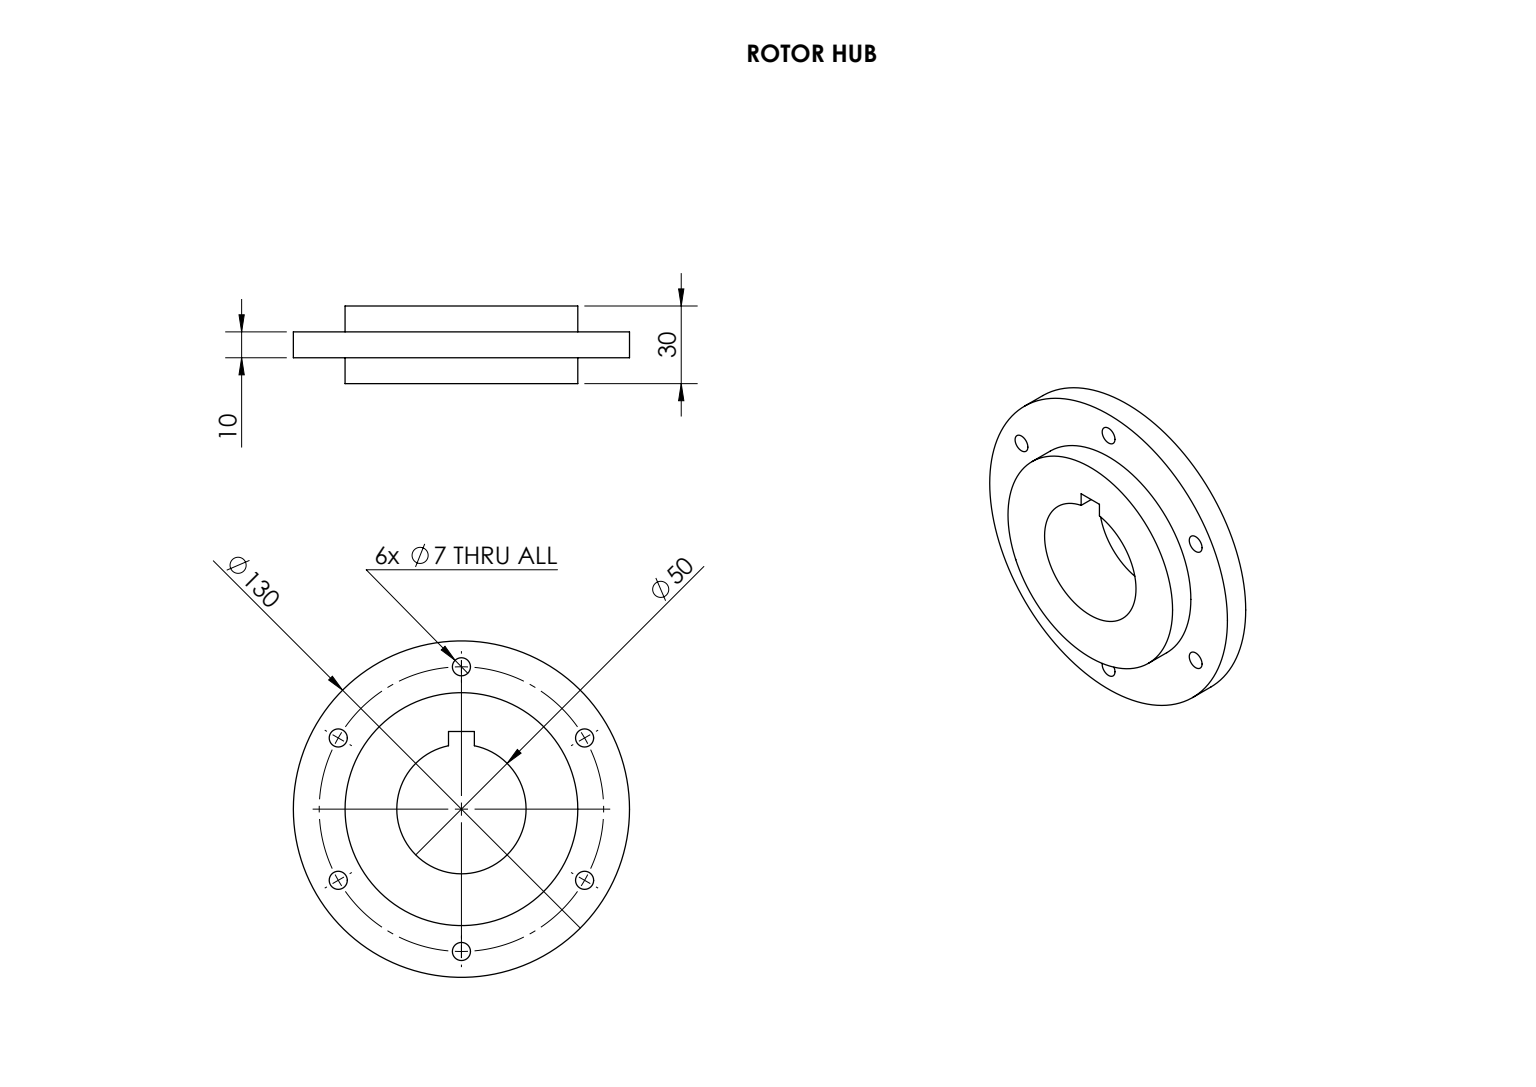
ISO-10303-21;
HEADER;
FILE_DESCRIPTION (('STEP AP214'),
    '1' );
FILE_NAME ('rotor hub.step',
    '2026-09-21T15:58:29',
    ( '' ),
    ( '' ),
    'SwSTEP 2.0',
    'SolidWorks 2026',
    '' );
FILE_SCHEMA (( 'AUTOMOTIVE_DESIGN' ));
ENDSEC;

DATA;
#23=ORIENTED_EDGE ( 'NONE', *, *, #7418, .F. ) ;
#62=ORIENTED_EDGE ( 'NONE', *, *, #28158, .F. ) ;
#132=EDGE_LOOP ( 'NONE', ( #17716, #15446, #15780, #32806 ) ) ;
#135=DIRECTION ( 'NONE',  ( 1.000000000000000000, 0.000000000000000000, 0.000000000000000000 ) ) ;
#170=EDGE_CURVE ( 'NONE', #35280, #21315, #27084, .T. ) ;
#178=CARTESIAN_POINT ( 'NONE',  ( 0.000000000000000000, 0.000000000000000000, -15.00000000000000000 ) ) ;
#209=EDGE_LOOP ( 'NONE', ( #36772, #14646 ) ) ;
#216=ORIENTED_EDGE ( 'NONE', *, *, #28158, .T. ) ;
#229=CARTESIAN_POINT ( 'NONE',  ( 0.000000000000000000, -55.00000000000000000, 5.000000000000000888 ) ) ;
#247=CARTESIAN_POINT ( 'NONE',  ( -47.63139720814438505, -27.49999999999955591, -5.000000000000000888 ) ) ;
#391=ORIENTED_EDGE ( 'NONE', *, *, #32304, .T. ) ;
#413=STYLED_ITEM ( 'NONE', ( #19324 ), #17045 ) ;
#421=ORIENTED_EDGE ( 'NONE', *, *, #12604, .F. ) ;
#524=VECTOR ( 'NONE', #22950, 1000.000000000000000 ) ;
#536=EDGE_CURVE ( 'NONE', #19811, #13357, #11783, .T. ) ;
#674=DIRECTION ( 'NONE',  ( 0.000000000000000000, 0.000000000000000000, 1.000000000000000000 ) ) ;
#679=EDGE_CURVE ( 'NONE', #31822, #13995, #25431, .T. ) ;
#680=FACE_OUTER_BOUND ( 'NONE', #28882, .T. ) ;
#743=DIRECTION ( 'NONE',  ( -1.000000000000000000, 0.000000000000000000, 0.000000000000000000 ) ) ;
#764=CARTESIAN_POINT ( 'NONE',  ( -5.000000000000000000, 24.49489742783178414, 15.00000000000000000 ) ) ;
#824=LINE ( 'NONE', #20902, #10192 ) ;
#838=DIRECTION ( 'NONE',  ( -1.000000000000000000, 0.000000000000000000, 0.000000000000000000 ) ) ;
#971=CARTESIAN_POINT ( 'NONE',  ( -45.00000000000000000, 0.000000000000000000, -15.00000000000000000 ) ) ;
#1002=EDGE_LOOP ( 'NONE', ( #30017, #31364, #12211, #17517 ) ) ;
#1009=ORIENTED_EDGE ( 'NONE', *, *, #1750, .F. ) ;
#1040=CARTESIAN_POINT ( 'NONE',  ( 0.000000000000000000, 55.00000000000000000, -15.00000000000000000 ) ) ;
#1174=DIRECTION ( 'NONE',  ( 1.000000000000000000, 0.000000000000000000, 0.000000000000000000 ) ) ;
#1179=DIRECTION ( 'NONE',  ( 1.000000000000000000, 0.000000000000000000, 0.000000000000000000 ) ) ;
#1187=ORIENTED_EDGE ( 'NONE', *, *, #32304, .F. ) ;
#1244=FACE_BOUND ( 'NONE', #25604, .T. ) ;
#1245=SURFACE_STYLE_USAGE ( .BOTH. , #13045 ) ;
#1283=ORIENTED_EDGE ( 'NONE', *, *, #14933, .F. ) ;
#1311=ORIENTED_EDGE ( 'NONE', *, *, #7418, .T. ) ;
#1329=ADVANCED_FACE ( 'NONE', ( #32145 ), #4233, .F. ) ;
#1402=FACE_OUTER_BOUND ( 'NONE', #32272, .T. ) ;
#1408=ORIENTED_EDGE ( 'NONE', *, *, #15156, .T. ) ;
#1419=PRESENTATION_STYLE_ASSIGNMENT (( #1245 ) ) ;
#1420=EDGE_LOOP ( 'NONE', ( #24774, #7913, #20426, #34060 ) ) ;
#1425=CARTESIAN_POINT ( 'NONE',  ( -4.999999999999999112, 24.49489742783178059, 15.00000000000000000 ) ) ;
#1484=VECTOR ( 'NONE', #4946, 1000.000000000000000 ) ;
#1578=CARTESIAN_POINT ( 'NONE',  ( -5.000000000000000000, 30.00000000000000355, -15.00000000000000000 ) ) ;
#1591=ORIENTED_EDGE ( 'NONE', *, *, #11289, .F. ) ;
#1630=( GEOMETRIC_REPRESENTATION_CONTEXT ( 3 ) GLOBAL_UNCERTAINTY_ASSIGNED_CONTEXT ( ( #8434 ) ) GLOBAL_UNIT_ASSIGNED_CONTEXT ( ( #30742, #18767, #10319 ) ) REPRESENTATION_CONTEXT ( 'NONE', 'WORKASPACE' ) );
#1650=PLANE ( 'NONE',  #21521 ) ;
#1656=DIRECTION ( 'NONE',  ( 0.000000000000000000, 0.000000000000000000, 1.000000000000000000 ) ) ;
#1674=VECTOR ( 'NONE', #17302, 1000.000000000000000 ) ;
#1750=EDGE_CURVE ( 'NONE', #19879, #6148, #24587, .T. ) ;
#1814=CARTESIAN_POINT ( 'NONE',  ( 0.000000000000000000, -55.00000000000000000, -5.000000000000000888 ) ) ;
#1817=CARTESIAN_POINT ( 'NONE',  ( -47.63139720814438505, -27.49999999999955591, -15.00000000000000000 ) ) ;
#1820=VERTEX_POINT ( 'NONE', #31898 ) ;
#1862=DIRECTION ( 'NONE',  ( -1.000000000000000000, 0.000000000000000000, 0.000000000000000000 ) ) ;
#1888=FILL_AREA_STYLE ('',( #4896 ) ) ;
#1909=DIRECTION ( 'NONE',  ( -0.000000000000000000, -0.000000000000000000, 1.000000000000000000 ) ) ;
#2009=DIRECTION ( 'NONE',  ( 1.000000000000000000, 0.000000000000000000, -0.000000000000000000 ) ) ;
#2013=PLANE ( 'NONE',  #17910 ) ;
#2051=CIRCLE ( 'NONE', #23596, 45.00000000000000000 ) ;
#2096=EDGE_LOOP ( 'NONE', ( #27715, #24224, #28476, #9643 ) ) ;
#2103=ORIENTED_EDGE ( 'NONE', *, *, #20963, .T. ) ;
#2104=AXIS2_PLACEMENT_3D ( 'NONE', #2399, #16446, #36696 ) ;
#2150=DIRECTION ( 'NONE',  ( 1.000000000000000000, 0.000000000000000000, 0.000000000000000000 ) ) ;
#2202=DIRECTION ( 'NONE',  ( 0.000000000000000000, 0.000000000000000000, 1.000000000000000000 ) ) ;
#2296=ORIENTED_EDGE ( 'NONE', *, *, #19769, .T. ) ;
#2368=EDGE_CURVE ( 'NONE', #24370, #17590, #4662, .T. ) ;
#2372=VERTEX_POINT ( 'NONE', #14928 ) ;
#2375=EDGE_CURVE ( 'NONE', #2372, #1820, #22821, .T. ) ;
#2399=CARTESIAN_POINT ( 'NONE',  ( 0.000000000000000000, 0.000000000000000000, 15.00000000000000000 ) ) ;
#2480=FACE_BOUND ( 'NONE', #36377, .T. ) ;
#2506=DIRECTION ( 'NONE',  ( -1.000000000000000000, 0.000000000000000000, 0.000000000000000000 ) ) ;
#2557=EDGE_CURVE ( 'NONE', #25534, #2372, #24485, .T. ) ;
#2569=ADVANCED_FACE ( 'NONE', ( #1402 ), #12824, .F. ) ;
#2602=VECTOR ( 'NONE', #10246, 1000.000000000000000 ) ;
#2627=( GEOMETRIC_REPRESENTATION_CONTEXT ( 3 ) GLOBAL_UNCERTAINTY_ASSIGNED_CONTEXT ( ( #4325 ) ) GLOBAL_UNIT_ASSIGNED_CONTEXT ( ( #7421, #26546, #3684 ) ) REPRESENTATION_CONTEXT ( 'NONE', 'WORKASPACE' ) );
#2635=ORIENTED_EDGE ( 'NONE', *, *, #31325, .F. ) ;
#2639=DIRECTION ( 'NONE',  ( -0.000000000000000000, -0.000000000000000000, -1.000000000000000000 ) ) ;
#2674=PRODUCT_DEFINITION ( 'UNKNOWN', '', #29130, #14421 ) ;
#2703=CYLINDRICAL_SURFACE ( 'NONE', #25764, 3.500000000000003109 ) ;
#2741=DIRECTION ( 'NONE',  ( 1.000000000000000000, 0.000000000000000000, 0.000000000000000000 ) ) ;
#2758=EDGE_CURVE ( 'NONE', #24629, #10920, #12743, .T. ) ;
#2891=VECTOR ( 'NONE', #27089, 1000.000000000000000 ) ;
#2947=DIRECTION ( 'NONE',  ( 1.000000000000000000, 0.000000000000000000, 0.000000000000000000 ) ) ;
#2982=CIRCLE ( 'NONE', #8366, 3.500000000000003109 ) ;
#3001=ORIENTED_EDGE ( 'NONE', *, *, #20598, .F. ) ;
#3037=ORIENTED_EDGE ( 'NONE', *, *, #5291, .T. ) ;
#3041=FACE_BOUND ( 'NONE', #30009, .T. ) ;
#3057=CARTESIAN_POINT ( 'NONE',  ( -51.13139720814438505, -27.49999999999955591, -15.00000000000000000 ) ) ;
#3059=ORIENTED_EDGE ( 'NONE', *, *, #2557, .F. ) ;
#3067=CARTESIAN_POINT ( 'NONE',  ( 44.13139720814418610, 27.49999999999988987, -5.000000000000000888 ) ) ;
#3157=CARTESIAN_POINT ( 'NONE',  ( -25.00000000000000000, 0.000000000000000000, 15.00000000000000000 ) ) ;
#3160=EDGE_CURVE ( 'NONE', #36052, #13357, #33221, .T. ) ;
#3172=EDGE_CURVE ( 'NONE', #35280, #29596, #27218, .T. ) ;
#3174=APPLICATION_CONTEXT ( 'automotive_design' ) ;
#3181=DIRECTION ( 'NONE',  ( 0.000000000000000000, 0.000000000000000000, 1.000000000000000000 ) ) ;
#3198=CARTESIAN_POINT ( 'NONE',  ( -47.63139720814380951, 27.50000000000055422, -5.000000000000000888 ) ) ;
#3241=DIRECTION ( 'NONE',  ( 0.000000000000000000, -0.000000000000000000, -1.000000000000000000 ) ) ;
#3281=EDGE_CURVE ( 'NONE', #17590, #24370, #24061, .T. ) ;
#3324=VERTEX_POINT ( 'NONE', #22732 ) ;
#3335=AXIS2_PLACEMENT_3D ( 'NONE', #13182, #24631, #33228 ) ;
#3356=ADVANCED_FACE ( 'NONE', ( #11815, #16738, #3041, #2480, #5479, #16905, #36978, #34524 ), #8469, .F. ) ;
#3417=DIRECTION ( 'NONE',  ( 1.000000000000000000, 0.000000000000000000, 0.000000000000000000 ) ) ;
#3427=COLOUR_RGB ( '', 0.08235294, 0.09019608, 0.10196078) ;
#3448=VERTEX_POINT ( 'NONE', #6941 ) ;
#3599=DIRECTION ( 'NONE',  ( 0.000000000000000000, 0.000000000000000000, 1.000000000000000000 ) ) ;
#3601=LINE ( 'NONE', #3057, #11251 ) ;
#3608=ORIENTED_EDGE ( 'NONE', *, *, #10532, .F. ) ;
#3673=CARTESIAN_POINT ( 'NONE',  ( -5.000000000000000000, 25.00000000000000000, 15.00000000000000000 ) ) ;
#3684=( NAMED_UNIT ( * ) SI_UNIT ( $, .STERADIAN. ) SOLID_ANGLE_UNIT ( ) );
#3692=CARTESIAN_POINT ( 'NONE',  ( -45.00000000000000000, 0.000000000000000000, 15.00000000000000000 ) ) ;
#3696=EDGE_CURVE ( 'NONE', #24370, #5854, #12082, .T. ) ;
#3717=DIRECTION ( 'NONE',  ( 1.000000000000000000, 0.000000000000000000, 0.000000000000000000 ) ) ;
#3725=DIRECTION ( 'NONE',  ( 0.000000000000000000, 0.000000000000000000, 1.000000000000000000 ) ) ;
#3769=ORIENTED_EDGE ( 'NONE', *, *, #32301, .T. ) ;
#3854=CARTESIAN_POINT ( 'NONE',  ( 0.000000000000000000, 0.000000000000000000, -15.00000000000000000 ) ) ;
#3882=EDGE_CURVE ( 'NONE', #4744, #14689, #24525, .T. ) ;
#3948=AXIS2_PLACEMENT_3D ( 'NONE', #178, #26255, #26610 ) ;
#3959=CIRCLE ( 'NONE', #20729, 3.500000000000003109 ) ;
#4002=VECTOR ( 'NONE', #29085, 1000.000000000000000 ) ;
#4077=EDGE_CURVE ( 'NONE', #3448, #10920, #10594, .T. ) ;
#4084=VECTOR ( 'NONE', #35649, 1000.000000000000000 ) ;
#4133=AXIS2_PLACEMENT_3D ( 'NONE', #9406, #15208, #3417 ) ;
#4185=EDGE_CURVE ( 'NONE', #25427, #11646, #25588, .T. ) ;
#4220=AXIS2_PLACEMENT_3D ( 'NONE', #28699, #9174, #743 ) ;
#4226=LINE ( 'NONE', #10576, #1484 ) ;
#4233=CYLINDRICAL_SURFACE ( 'NONE', #13387, 25.00000000000000000 ) ;
#4250=DIRECTION ( 'NONE',  ( 1.000000000000000000, 0.000000000000000000, 0.000000000000000000 ) ) ;
#4325=UNCERTAINTY_MEASURE_WITH_UNIT (LENGTH_MEASURE( 1.000000000000000082E-05 ), #7421, 'distance_accuracy_value', 'NONE');
#4383=CYLINDRICAL_SURFACE ( 'NONE', #11462, 25.00000000000000000 ) ;
#4432=CARTESIAN_POINT ( 'NONE',  ( 47.63139720814418610, 27.49999999999988987, -15.00000000000000000 ) ) ;
#4440=CARTESIAN_POINT ( 'NONE',  ( 3.500000000000000888, -55.00000000000000000, -15.00000000000000000 ) ) ;
#4478=VERTEX_POINT ( 'NONE', #22181 ) ;
#4500=CIRCLE ( 'NONE', #20064, 3.500000000000000888 ) ;
#4514=EDGE_LOOP ( 'NONE', ( #5305, #3608, #4752, #1408 ) ) ;
#4561=EDGE_CURVE ( 'NONE', #25776, #5222, #16511, .T. ) ;
#4602=ORIENTED_EDGE ( 'NONE', *, *, #13796, .T. ) ;
#4609=DIRECTION ( 'NONE',  ( 0.000000000000000000, 0.000000000000000000, 1.000000000000000000 ) ) ;
#4617=VECTOR ( 'NONE', #35577, 1000.000000000000000 ) ;
#4662=CIRCLE ( 'NONE', #22641, 3.500000000000003109 ) ;
#4744=VERTEX_POINT ( 'NONE', #9944 ) ;
#4752=ORIENTED_EDGE ( 'NONE', *, *, #35183, .T. ) ;
#4757=ORIENTED_EDGE ( 'NONE', *, *, #10532, .T. ) ;
#4765=FACE_OUTER_BOUND ( 'NONE', #4997, .T. ) ;
#4783=EDGE_CURVE ( 'NONE', #30464, #18023, #13532, .T. ) ;
#4848=FACE_BOUND ( 'NONE', #18275, .T. ) ;
#4860=AXIS2_PLACEMENT_3D ( 'NONE', #14407, #26015, #135 ) ;
#4896=FILL_AREA_STYLE_COLOUR ( '', #3427 ) ;
#4915=DIRECTION ( 'NONE',  ( 1.000000000000000000, 0.000000000000000000, 0.000000000000000000 ) ) ;
#4921=DIRECTION ( 'NONE',  ( 1.000000000000000000, 0.000000000000000000, 0.000000000000000000 ) ) ;
#4946=DIRECTION ( 'NONE',  ( -0.000000000000000000, -0.000000000000000000, 1.000000000000000000 ) ) ;
#4997=EDGE_LOOP ( 'NONE', ( #31009, #30211, #12672, #1591 ) ) ;
#4998=ORIENTED_EDGE ( 'NONE', *, *, #3172, .T. ) ;
#5065=SHAPE_REPRESENTATION_RELATIONSHIP ( 'NONE' , 'NONE' ,  #33474, #17045 ) ;
#5086=CARTESIAN_POINT ( 'NONE',  ( 25.00000000000000000, 3.061616997868383043E-15, 15.00000000000000000 ) ) ;
#5210=CARTESIAN_POINT ( 'NONE',  ( 0.000000000000000000, 0.000000000000000000, 5.000000000000000000 ) ) ;
#5222=VERTEX_POINT ( 'NONE', #26891 ) ;
#5259=EDGE_CURVE ( 'NONE', #10522, #31822, #7379, .T. ) ;
#5275=ORIENTED_EDGE ( 'NONE', *, *, #12604, .T. ) ;
#5291=EDGE_CURVE ( 'NONE', #31944, #11785, #16372, .T. ) ;
#5305=ORIENTED_EDGE ( 'NONE', *, *, #26190, .F. ) ;
#5392=CARTESIAN_POINT ( 'NONE',  ( -5.000000000000000000, 30.00000000000000355, -15.00000000000000000 ) ) ;
#5416=AXIS2_PLACEMENT_3D ( 'NONE', #229, #23120, #28913 ) ;
#5479=FACE_BOUND ( 'NONE', #29963, .T. ) ;
#5592=DIRECTION ( 'NONE',  ( -0.000000000000000000, -0.000000000000000000, 1.000000000000000000 ) ) ;
#5694=AXIS2_PLACEMENT_3D ( 'NONE', #32993, #7307, #13120 ) ;
#5730=CARTESIAN_POINT ( 'NONE',  ( 0.000000000000000000, 0.000000000000000000, 15.00000000000000000 ) ) ;
#5761=CARTESIAN_POINT ( 'NONE',  ( -51.13139720814380951, 27.50000000000055422, -5.000000000000000888 ) ) ;
#5846=DIRECTION ( 'NONE',  ( 0.000000000000000000, 0.000000000000000000, 1.000000000000000000 ) ) ;
#5854=VERTEX_POINT ( 'NONE', #28984 ) ;
#5899=CARTESIAN_POINT ( 'NONE',  ( 5.000000000000000000, 24.49489742783178414, -15.00000000000000000 ) ) ;
#5910=( LENGTH_UNIT ( ) NAMED_UNIT ( * ) SI_UNIT ( .MILLI., .METRE. ) );
#6012=ORIENTED_EDGE ( 'NONE', *, *, #2758, .F. ) ;
#6044=DIRECTION ( 'NONE',  ( 1.000000000000000000, 0.000000000000000000, 0.000000000000000000 ) ) ;
#6073=VECTOR ( 'NONE', #25857, 1000.000000000000000 ) ;
#6092=CARTESIAN_POINT ( 'NONE',  ( -65.00000000000000000, 0.000000000000000000, 5.000000000000000000 ) ) ;
#6148=VERTEX_POINT ( 'NONE', #32743 ) ;
#6412=DIRECTION ( 'NONE',  ( 1.000000000000000000, 0.000000000000000000, 0.000000000000000000 ) ) ;
#6432=AXIS2_PLACEMENT_3D ( 'NONE', #6988, #10187, #29863 ) ;
#6489=ORIENTED_EDGE ( 'NONE', *, *, #19945, .T. ) ;
#6491=DIRECTION ( 'NONE',  ( 1.000000000000000000, 0.000000000000000000, 0.000000000000000000 ) ) ;
#6588=EDGE_CURVE ( 'NONE', #3448, #14395, #16778, .T. ) ;
#6795=COLOUR_RGB ( '', 0.08235294, 0.09019608, 0.10196078) ;
#6813=FACE_OUTER_BOUND ( 'NONE', #132, .T. ) ;
#6842=DIRECTION ( 'NONE',  ( 1.000000000000000000, 0.000000000000000000, 0.000000000000000000 ) ) ;
#6873=EDGE_CURVE ( 'NONE', #11785, #11646, #22180, .T. ) ;
#6941=CARTESIAN_POINT ( 'NONE',  ( 51.13139720814400846, -27.50000000000022737, -5.000000000000000888 ) ) ;
#6956=DIRECTION ( 'NONE',  ( 1.000000000000000000, 0.000000000000000000, 0.000000000000000000 ) ) ;
#6978=DIRECTION ( 'NONE',  ( 0.000000000000000000, 0.000000000000000000, 1.000000000000000000 ) ) ;
#6986=DIRECTION ( 'NONE',  ( 1.000000000000000000, 0.000000000000000000, 0.000000000000000000 ) ) ;
#6988=CARTESIAN_POINT ( 'NONE',  ( 0.000000000000000000, 0.000000000000000000, -5.000000000000000000 ) ) ;
#7014=DIRECTION ( 'NONE',  ( -1.000000000000000000, 0.000000000000000000, 0.000000000000000000 ) ) ;
#7071=CYLINDRICAL_SURFACE ( 'NONE', #28018, 3.500000000000003109 ) ;
#7095=CARTESIAN_POINT ( 'NONE',  ( -47.63139720814380951, 27.50000000000055422, -15.00000000000000000 ) ) ;
#7159=AXIS2_PLACEMENT_3D ( 'NONE', #5210, #1656, #27882 ) ;
#7183=CIRCLE ( 'NONE', #28131, 45.00000000000000000 ) ;
#7246=ORIENTED_EDGE ( 'NONE', *, *, #34520, .T. ) ;
#7307=DIRECTION ( 'NONE',  ( 0.000000000000000000, 0.000000000000000000, 1.000000000000000000 ) ) ;
#7321=UNCERTAINTY_MEASURE_WITH_UNIT (LENGTH_MEASURE( 1.000000000000000082E-05 ), #5910, 'distance_accuracy_value', 'NONE');
#7379=LINE ( 'NONE', #12228, #18359 ) ;
#7407=DIRECTION ( 'NONE',  ( 0.000000000000000000, 0.000000000000000000, -1.000000000000000000 ) ) ;
#7418=EDGE_CURVE ( 'NONE', #31822, #2372, #16028, .T. ) ;
#7421=( LENGTH_UNIT ( ) NAMED_UNIT ( * ) SI_UNIT ( .MILLI., .METRE. ) );
#7528=DIRECTION ( 'NONE',  ( -0.000000000000000000, 0.000000000000000000, 1.000000000000000000 ) ) ;
#7575=AXIS2_PLACEMENT_3D ( 'NONE', #24426, #6978, #1179 ) ;
#7647=CYLINDRICAL_SURFACE ( 'NONE', #2104, 45.00000000000000000 ) ;
#7709=CYLINDRICAL_SURFACE ( 'NONE', #21484, 25.00000000000000000 ) ;
#7740=CARTESIAN_POINT ( 'NONE',  ( 0.000000000000000000, 55.00000000000000000, -5.000000000000000888 ) ) ;
#7764=CARTESIAN_POINT ( 'NONE',  ( 5.000000000000000000, 24.49489742783178414, 15.00000000000000000 ) ) ;
#7773=AXIS2_PLACEMENT_3D ( 'NONE', #7095, #12882, #18542 ) ;
#7830=DIRECTION ( 'NONE',  ( 0.000000000000000000, 0.000000000000000000, 1.000000000000000000 ) ) ;
#7859=EDGE_CURVE ( 'NONE', #11646, #11785, #16773, .T. ) ;
#7913=ORIENTED_EDGE ( 'NONE', *, *, #20003, .T. ) ;
#7971=DIRECTION ( 'NONE',  ( 1.000000000000000000, 0.000000000000000000, 0.000000000000000000 ) ) ;
#7994=DIRECTION ( 'NONE',  ( 1.000000000000000000, 0.000000000000000000, 0.000000000000000000 ) ) ;
#8033=AXIS2_PLACEMENT_3D ( 'NONE', #20629, #3599, #6044 ) ;
#8044=EDGE_CURVE ( 'NONE', #21315, #26861, #31149, .T. ) ;
#8098=DIRECTION ( 'NONE',  ( -0.000000000000000000, 0.000000000000000000, 1.000000000000000000 ) ) ;
#8104=AXIS2_PLACEMENT_3D ( 'NONE', #35168, #20703, #9655 ) ;
#8113=ADVANCED_FACE ( 'NONE', ( #20604 ), #17443, .T. ) ;
#8219=CLOSED_SHELL ( 'NONE', ( #14021, #22878, #20690, #14478, #10904, #2569, #18517, #22051, #1329, #28849, #22091, #35522, #14922, #15263, #17435, #11394, #34187, #8591, #30019, #13997, #3356, #8113, #17566, #19990, #13254, #27020, #30785, #29252 ) ) ;
#8250=CARTESIAN_POINT ( 'NONE',  ( 3.500000000000000888, 55.00000000000000000, 5.000000000000000888 ) ) ;
#8366=AXIS2_PLACEMENT_3D ( 'NONE', #18502, #10408, #4250 ) ;
#8384=DIRECTION ( 'NONE',  ( 0.000000000000000000, 0.000000000000000000, 1.000000000000000000 ) ) ;
#8434=UNCERTAINTY_MEASURE_WITH_UNIT (LENGTH_MEASURE( 1.000000000000000082E-05 ), #30742, 'distance_accuracy_value', 'NONE');
#8469=PLANE ( 'NONE',  #19276 ) ;
#8537=EDGE_CURVE ( 'NONE', #25534, #35280, #16235, .T. ) ;
#8591=ADVANCED_FACE ( 'NONE', ( #34836 ), #9132, .T. ) ;
#8630=LINE ( 'NONE', #28317, #33793 ) ;
#8642=ORIENTED_EDGE ( 'NONE', *, *, #8739, .T. ) ;
#8658=EDGE_LOOP ( 'NONE', ( #27899, #10390 ) ) ;
#8702=AXIS2_PLACEMENT_3D ( 'NONE', #27436, #30054, #24243 ) ;
#8722=CARTESIAN_POINT ( 'NONE',  ( 25.00000000000000000, 3.061616997868383043E-15, -15.00000000000000000 ) ) ;
#8739=EDGE_CURVE ( 'NONE', #13777, #14961, #20102, .T. ) ;
#8762=ORIENTED_EDGE ( 'NONE', *, *, #19494, .T. ) ;
#8880=AXIS2_PLACEMENT_3D ( 'NONE', #15616, #13335, #4915 ) ;
#8896=CARTESIAN_POINT ( 'NONE',  ( 0.000000000000000000, 0.000000000000000000, 0.000000000000000000 ) ) ;
#8913=DIRECTION ( 'NONE',  ( -0.000000000000000000, -0.000000000000000000, -1.000000000000000000 ) ) ;
#8924=ORIENTED_EDGE ( 'NONE', *, *, #20598, .T. ) ;
#9008=ORIENTED_EDGE ( 'NONE', *, *, #27912, .F. ) ;
#9095=ORIENTED_EDGE ( 'NONE', *, *, #32301, .F. ) ;
#9111=CARTESIAN_POINT ( 'NONE',  ( 0.000000000000000000, 0.000000000000000000, -15.00000000000000000 ) ) ;
#9128=AXIS2_PLACEMENT_3D ( 'NONE', #16301, #13465, #1862 ) ;
#9132=PLANE ( 'NONE',  #23422 ) ;
#9174=DIRECTION ( 'NONE',  ( -0.000000000000000000, -0.000000000000000000, -1.000000000000000000 ) ) ;
#9226=ORIENTED_EDGE ( 'NONE', *, *, #8044, .T. ) ;
#9264=DIRECTION ( 'NONE',  ( -0.000000000000000000, -0.000000000000000000, 1.000000000000000000 ) ) ;
#9406=CARTESIAN_POINT ( 'NONE',  ( 0.000000000000000000, 0.000000000000000000, 5.000000000000000000 ) ) ;
#9504=DIRECTION ( 'NONE',  ( 1.000000000000000000, 0.000000000000000000, 0.000000000000000000 ) ) ;
#9585=EDGE_CURVE ( 'NONE', #20938, #36052, #27332, .T. ) ;
#9595=LINE ( 'NONE', #23647, #34378 ) ;
#9643=ORIENTED_EDGE ( 'NONE', *, *, #7859, .T. ) ;
#9655=DIRECTION ( 'NONE',  ( 1.000000000000000000, 0.000000000000000000, 0.000000000000000000 ) ) ;
#9676=ORIENTED_EDGE ( 'NONE', *, *, #30500, .T. ) ;
#9688=ORIENTED_EDGE ( 'NONE', *, *, #13106, .F. ) ;
#9800=ORIENTED_EDGE ( 'NONE', *, *, #2758, .T. ) ;
#9836=CARTESIAN_POINT ( 'NONE',  ( 5.000000000000000000, 25.00000000000000000, -15.00000000000000000 ) ) ;
#9907=CARTESIAN_POINT ( 'NONE',  ( 45.00000000000000711, 5.510910596163091133E-15, 5.000000000000000000 ) ) ;
#9930=DIRECTION ( 'NONE',  ( 0.000000000000000000, -0.000000000000000000, 1.000000000000000000 ) ) ;
#9944=CARTESIAN_POINT ( 'NONE',  ( 65.00000000000000000, 7.960204194457797252E-15, -5.000000000000000000 ) ) ;
#9946=ORIENTED_EDGE ( 'NONE', *, *, #13106, .T. ) ;
#10099=ORIENTED_EDGE ( 'NONE', *, *, #4077, .T. ) ;
#10187=DIRECTION ( 'NONE',  ( 0.000000000000000000, 0.000000000000000000, 1.000000000000000000 ) ) ;
#10192=VECTOR ( 'NONE', #12237, 1000.000000000000000 ) ;
#10222=PLANE ( 'NONE',  #30953 ) ;
#10246=DIRECTION ( 'NONE',  ( -0.000000000000000000, 1.000000000000000000, 0.000000000000000000 ) ) ;
#10319=( NAMED_UNIT ( * ) SI_UNIT ( $, .STERADIAN. ) SOLID_ANGLE_UNIT ( ) );
#10363=EDGE_LOOP ( 'NONE', ( #34270, #9226, #62, #34153 ) ) ;
#10390=ORIENTED_EDGE ( 'NONE', *, *, #2368, .T. ) ;
#10399=PRODUCT ( 'rotor hub', 'rotor hub', '', ( #12666 ) ) ;
#10408=DIRECTION ( 'NONE',  ( 0.000000000000000000, 0.000000000000000000, 1.000000000000000000 ) ) ;
#10450=DIRECTION ( 'NONE',  ( 1.000000000000000000, 0.000000000000000000, -0.000000000000000000 ) ) ;
#10522=VERTEX_POINT ( 'NONE', #18345 ) ;
#10532=EDGE_CURVE ( 'NONE', #14697, #30372, #16441, .T. ) ;
#10538=FACE_OUTER_BOUND ( 'NONE', #16439, .T. ) ;
#10576=CARTESIAN_POINT ( 'NONE',  ( -3.500000000000000888, -55.00000000000000000, -15.00000000000000000 ) ) ;
#10594=LINE ( 'NONE', #16951, #19699 ) ;
#10610=SHAPE_DEFINITION_REPRESENTATION ( #17857, #33474 ) ;
#10619=EDGE_CURVE ( 'NONE', #25427, #31944, #32622, .T. ) ;
#10656=FACE_OUTER_BOUND ( 'NONE', #13476, .T. ) ;
#10705=SURFACE_SIDE_STYLE ('',( #13492 ) ) ;
#10806=DIRECTION ( 'NONE',  ( 1.000000000000000000, 0.000000000000000000, 0.000000000000000000 ) ) ;
#10836=FACE_OUTER_BOUND ( 'NONE', #29415, .T. ) ;
#10904=ADVANCED_FACE ( 'NONE', ( #4765 ), #12619, .F. ) ;
#10920=VERTEX_POINT ( 'NONE', #35514 ) ;
#10951=CARTESIAN_POINT ( 'NONE',  ( 47.63139720814418610, 27.49999999999988987, -5.000000000000000888 ) ) ;
#11129=EDGE_CURVE ( 'NONE', #10522, #25534, #14645, .T. ) ;
#11189=EDGE_CURVE ( 'NONE', #20938, #19811, #3601, .T. ) ;
#11236=DIRECTION ( 'NONE',  ( 0.000000000000000000, 0.000000000000000000, 1.000000000000000000 ) ) ;
#11251=VECTOR ( 'NONE', #31523, 1000.000000000000000 ) ;
#11254=ORIENTED_EDGE ( 'NONE', *, *, #36027, .T. ) ;
#11257=EDGE_LOOP ( 'NONE', ( #13857, #17632, #5275, #9946 ) ) ;
#11289=EDGE_CURVE ( 'NONE', #4478, #25776, #27394, .T. ) ;
#11337=FACE_OUTER_BOUND ( 'NONE', #11456, .T. ) ;
#11394=ADVANCED_FACE ( 'NONE', ( #33760 ), #7709, .F. ) ;
#11437=CARTESIAN_POINT ( 'NONE',  ( 0.000000000000000000, 0.000000000000000000, 5.000000000000000000 ) ) ;
#11441=DIRECTION ( 'NONE',  ( 1.000000000000000000, 0.000000000000000000, 0.000000000000000000 ) ) ;
#11442=ORIENTED_EDGE ( 'NONE', *, *, #12384, .F. ) ;
#11454=DIRECTION ( 'NONE',  ( 0.000000000000000000, 0.000000000000000000, 1.000000000000000000 ) ) ;
#11456=EDGE_LOOP ( 'NONE', ( #23334, #18031, #9800, #33838 ) ) ;
#11462=AXIS2_PLACEMENT_3D ( 'NONE', #35898, #32686, #7014 ) ;
#11618=CARTESIAN_POINT ( 'NONE',  ( -5.000000000000000000, 30.00000000000000355, -15.00000000000000000 ) ) ;
#11646=VERTEX_POINT ( 'NONE', #29410 ) ;
#11741=AXIS2_PLACEMENT_3D ( 'NONE', #247, #34591, #29121 ) ;
#11752=ORIENTED_EDGE ( 'NONE', *, *, #2375, .T. ) ;
#11783=CIRCLE ( 'NONE', #32758, 3.500000000000003109 ) ;
#11785=VERTEX_POINT ( 'NONE', #9907 ) ;
#11815=FACE_BOUND ( 'NONE', #8658, .T. ) ;
#11961=AXIS2_PLACEMENT_3D ( 'NONE', #1814, #13241, #36119 ) ;
#12082=LINE ( 'NONE', #23543, #6073 ) ;
#12211=ORIENTED_EDGE ( 'NONE', *, *, #3160, .T. ) ;
#12228=CARTESIAN_POINT ( 'NONE',  ( -5.000000000000000000, 25.00000000000000000, -15.00000000000000000 ) ) ;
#12237=DIRECTION ( 'NONE',  ( -0.000000000000000000, -0.000000000000000000, -1.000000000000000000 ) ) ;
#12306=AXIS2_PLACEMENT_3D ( 'NONE', #10951, #4609, #22907 ) ;
#12336=CIRCLE ( 'NONE', #7575, 3.500000000000003109 ) ;
#12384=EDGE_CURVE ( 'NONE', #21315, #22186, #25749, .T. ) ;
#12405=EDGE_CURVE ( 'NONE', #18518, #21193, #14976, .T. ) ;
#12446=AXIS2_PLACEMENT_3D ( 'NONE', #1040, #32916, #6491 ) ;
#12486=AXIS2_PLACEMENT_3D ( 'NONE', #7740, #30604, #4921 ) ;
#12574=AXIS2_PLACEMENT_3D ( 'NONE', #11437, #3181, #17802 ) ;
#12604=EDGE_CURVE ( 'NONE', #25787, #14689, #824, .T. ) ;
#12619=CYLINDRICAL_SURFACE ( 'NONE', #8702, 3.500000000000003109 ) ;
#12657=ORIENTED_EDGE ( 'NONE', *, *, #9585, .F. ) ;
#12666=PRODUCT_CONTEXT ( 'NONE', #3174, 'mechanical' ) ;
#12672=ORIENTED_EDGE ( 'NONE', *, *, #16828, .T. ) ;
#12674=DIRECTION ( 'NONE',  ( 0.000000000000000000, -0.000000000000000000, 1.000000000000000000 ) ) ;
#12743=CIRCLE ( 'NONE', #22964, 3.500000000000003109 ) ;
#12808=AXIS2_PLACEMENT_3D ( 'NONE', #21595, #33395, #6956 ) ;
#12818=DIRECTION ( 'NONE',  ( -0.000000000000000000, -0.000000000000000000, -1.000000000000000000 ) ) ;
#12824=CYLINDRICAL_SURFACE ( 'NONE', #12446, 3.500000000000000888 ) ;
#12882=DIRECTION ( 'NONE',  ( -0.000000000000000000, -0.000000000000000000, 1.000000000000000000 ) ) ;
#12887=CARTESIAN_POINT ( 'NONE',  ( -3.500000000000000888, 55.00000000000000000, 5.000000000000000888 ) ) ;
#12924=VERTEX_POINT ( 'NONE', #5899 ) ;
#13017=ORIENTED_EDGE ( 'NONE', *, *, #15156, .F. ) ;
#13030=VECTOR ( 'NONE', #24746, 1000.000000000000000 ) ;
#13043=CIRCLE ( 'NONE', #6432, 65.00000000000000000 ) ;
#13045=SURFACE_SIDE_STYLE ('',( #35749 ) ) ;
#13052=FACE_OUTER_BOUND ( 'NONE', #27825, .T. ) ;
#13072=DIRECTION ( 'NONE',  ( 1.000000000000000000, 0.000000000000000000, 0.000000000000000000 ) ) ;
#13079=AXIS2_PLACEMENT_3D ( 'NONE', #27365, #9930, #33167 ) ;
#13106=EDGE_CURVE ( 'NONE', #14689, #4744, #13043, .T. ) ;
#13119=AXIS2_PLACEMENT_3D ( 'NONE', #23033, #11236, #22684 ) ;
#13120=DIRECTION ( 'NONE',  ( 1.000000000000000000, 0.000000000000000000, 0.000000000000000000 ) ) ;
#13174=CARTESIAN_POINT ( 'NONE',  ( -44.13139720814437794, -27.49999999999955591, -15.00000000000000000 ) ) ;
#13182=CARTESIAN_POINT ( 'NONE',  ( 47.63139720814418610, 27.49999999999988987, 5.000000000000000888 ) ) ;
#13203=CARTESIAN_POINT ( 'NONE',  ( 47.63139720814400846, -27.50000000000022737, -5.000000000000000888 ) ) ;
#13216=ORIENTED_EDGE ( 'NONE', *, *, #19835, .T. ) ;
#13238=DIRECTION ( 'NONE',  ( -0.000000000000000000, -0.000000000000000000, 1.000000000000000000 ) ) ;
#13241=DIRECTION ( 'NONE',  ( 0.000000000000000000, 0.000000000000000000, 1.000000000000000000 ) ) ;
#13254=ADVANCED_FACE ( 'NONE', ( #10538 ), #21983, .F. ) ;
#13268=EDGE_CURVE ( 'NONE', #3324, #24335, #16104, .T. ) ;
#13292=DIRECTION ( 'NONE',  ( 0.000000000000000000, 0.000000000000000000, 1.000000000000000000 ) ) ;
#13335=DIRECTION ( 'NONE',  ( 0.000000000000000000, 0.000000000000000000, 1.000000000000000000 ) ) ;
#13340=DIRECTION ( 'NONE',  ( 0.000000000000000000, 0.000000000000000000, 1.000000000000000000 ) ) ;
#13357=VERTEX_POINT ( 'NONE', #20443 ) ;
#13358=ORIENTED_EDGE ( 'NONE', *, *, #4783, .F. ) ;
#13379=MECHANICAL_DESIGN_GEOMETRIC_PRESENTATION_REPRESENTATION('',(#26574),#2627);
#13387=AXIS2_PLACEMENT_3D ( 'NONE', #15662, #12818, #838 ) ;
#13396=AXIS2_PLACEMENT_3D ( 'NONE', #36689, #8384, #2741 ) ;
#13439=DIRECTION ( 'NONE',  ( 0.000000000000000000, 0.000000000000000000, 1.000000000000000000 ) ) ;
#13465=DIRECTION ( 'NONE',  ( -0.000000000000000000, -0.000000000000000000, -1.000000000000000000 ) ) ;
#13469=CARTESIAN_POINT ( 'NONE',  ( -51.13139720814438505, -27.49999999999955591, 5.000000000000000888 ) ) ;
#13476=EDGE_LOOP ( 'NONE', ( #31447, #9676 ) ) ;
#13478=EDGE_LOOP ( 'NONE', ( #19906, #35429 ) ) ;
#13492=SURFACE_STYLE_FILL_AREA ( #1888 ) ;
#13532=CIRCLE ( 'NONE', #27907, 45.00000000000000000 ) ;
#13551=DIRECTION ( 'NONE',  ( -0.000000000000000000, -0.000000000000000000, -1.000000000000000000 ) ) ;
#13727=AXIS2_PLACEMENT_3D ( 'NONE', #24282, #24489, #6842 ) ;
#13777=VERTEX_POINT ( 'NONE', #8250 ) ;
#13796=EDGE_CURVE ( 'NONE', #6148, #19879, #35878, .T. ) ;
#13844=EDGE_LOOP ( 'NONE', ( #391, #34050 ) ) ;
#13854=CARTESIAN_POINT ( 'NONE',  ( 5.000000000000000000, 24.49489742783178414, 15.00000000000000000 ) ) ;
#13857=ORIENTED_EDGE ( 'NONE', *, *, #19494, .F. ) ;
#13947=DIRECTION ( 'NONE',  ( -0.000000000000000000, 0.000000000000000000, 1.000000000000000000 ) ) ;
#13995=VERTEX_POINT ( 'NONE', #19105 ) ;
#13997=ADVANCED_FACE ( 'NONE', ( #19274, #30529, #27524, #30131, #27875, #4848, #30690, #16278 ), #1650, .T. ) ;
#14021=ADVANCED_FACE ( 'NONE', ( #10836 ), #32774, .F. ) ;
#14114=AXIS2_PLACEMENT_3D ( 'NONE', #36808, #31538, #2506 ) ;
#14189=ORIENTED_EDGE ( 'NONE', *, *, #3696, .T. ) ;
#14251=CARTESIAN_POINT ( 'NONE',  ( 47.63139720814400846, -27.50000000000022737, -5.000000000000000888 ) ) ;
#14254=DIRECTION ( 'NONE',  ( -1.000000000000000000, 0.000000000000000000, 0.000000000000000000 ) ) ;
#14256=ORIENTED_EDGE ( 'NONE', *, *, #536, .T. ) ;
#14284=DIRECTION ( 'NONE',  ( 1.000000000000000000, 0.000000000000000000, -0.000000000000000000 ) ) ;
#14374=CARTESIAN_POINT ( 'NONE',  ( -5.000000000000000000, 30.00000000000000355, 15.00000000000000000 ) ) ;
#14395=VERTEX_POINT ( 'NONE', #32924 ) ;
#14407=CARTESIAN_POINT ( 'NONE',  ( 0.000000000000000000, 0.000000000000000000, 15.00000000000000000 ) ) ;
#14421=PRODUCT_DEFINITION_CONTEXT ( 'detailed design', #20687, 'design' ) ;
#14451=ORIENTED_EDGE ( 'NONE', *, *, #4561, .T. ) ;
#14465=ORIENTED_EDGE ( 'NONE', *, *, #11129, .T. ) ;
#14478=ADVANCED_FACE ( 'NONE', ( #11337 ), #2703, .F. ) ;
#14544=DIRECTION ( 'NONE',  ( 1.000000000000000000, 0.000000000000000000, 0.000000000000000000 ) ) ;
#14583=EDGE_LOOP ( 'NONE', ( #19347, #1311, #3059, #28096 ) ) ;
#14645=LINE ( 'NONE', #764, #1674 ) ;
#14646=ORIENTED_EDGE ( 'NONE', *, *, #536, .F. ) ;
#14689=VERTEX_POINT ( 'NONE', #19151 ) ;
#14694=( NAMED_UNIT ( * ) PLANE_ANGLE_UNIT ( ) SI_UNIT ( $, .RADIAN. ) );
#14697=VERTEX_POINT ( 'NONE', #22488 ) ;
#14709=ORIENTED_EDGE ( 'NONE', *, *, #2375, .F. ) ;
#14922=ADVANCED_FACE ( 'NONE', ( #18717, #10656 ), #2013, .T. ) ;
#14928=CARTESIAN_POINT ( 'NONE',  ( -5.000000000000000000, 30.00000000000000355, 15.00000000000000000 ) ) ;
#14933=EDGE_CURVE ( 'NONE', #37029, #25787, #29272, .T. ) ;
#14944=PLANE ( 'NONE',  #27519 ) ;
#14961=VERTEX_POINT ( 'NONE', #12887 ) ;
#14976=CIRCLE ( 'NONE', #11961, 3.500000000000000888 ) ;
#15038=CARTESIAN_POINT ( 'NONE',  ( 45.00000000000000000, 5.510910596163089556E-15, 15.00000000000000000 ) ) ;
#15141=DIRECTION ( 'NONE',  ( 1.000000000000000000, 0.000000000000000000, 0.000000000000000000 ) ) ;
#15147=EDGE_LOOP ( 'NONE', ( #14709, #23, #28139, #6489 ) ) ;
#15156=EDGE_CURVE ( 'NONE', #18023, #30464, #7183, .T. ) ;
#15208=DIRECTION ( 'NONE',  ( 0.000000000000000000, 0.000000000000000000, 1.000000000000000000 ) ) ;
#15231=ORIENTED_EDGE ( 'NONE', *, *, #12405, .T. ) ;
#15263=ADVANCED_FACE ( 'NONE', ( #680, #1244 ), #14944, .F. ) ;
#15332=FACE_OUTER_BOUND ( 'NONE', #4514, .T. ) ;
#15397=EDGE_CURVE ( 'NONE', #13357, #19811, #2982, .T. ) ;
#15446=ORIENTED_EDGE ( 'NONE', *, *, #26190, .T. ) ;
#15517=EDGE_CURVE ( 'NONE', #4478, #23649, #34595, .T. ) ;
#15545=ORIENTED_EDGE ( 'NONE', *, *, #8537, .F. ) ;
#15616=CARTESIAN_POINT ( 'NONE',  ( 0.000000000000000000, 0.000000000000000000, 15.00000000000000000 ) ) ;
#15647=DIRECTION ( 'NONE',  ( 1.000000000000000000, 0.000000000000000000, 0.000000000000000000 ) ) ;
#15662=CARTESIAN_POINT ( 'NONE',  ( 0.000000000000000000, 0.000000000000000000, 15.00000000000000000 ) ) ;
#15767=CYLINDRICAL_SURFACE ( 'NONE', #12808, 3.500000000000000888 ) ;
#15780=ORIENTED_EDGE ( 'NONE', *, *, #4783, .T. ) ;
#15963=EDGE_LOOP ( 'NONE', ( #26804, #4998, #2635, #14465 ) ) ;
#16028=LINE ( 'NONE', #1578, #37086 ) ;
#16104=CIRCLE ( 'NONE', #12486, 3.500000000000000888 ) ;
#16111=CARTESIAN_POINT ( 'NONE',  ( -3.500000000000000888, -55.00000000000000000, -5.000000000000000888 ) ) ;
#16120=DIRECTION ( 'NONE',  ( 0.000000000000000000, 0.000000000000000000, 1.000000000000000000 ) ) ;
#16127=CARTESIAN_POINT ( 'NONE',  ( 3.500000000000000888, -55.00000000000000000, -5.000000000000000888 ) ) ;
#16235=CIRCLE ( 'NONE', #4860, 25.00000000000000000 ) ;
#16278=FACE_BOUND ( 'NONE', #28835, .T. ) ;
#16301=CARTESIAN_POINT ( 'NONE',  ( 0.000000000000000000, 0.000000000000000000, 5.000000000000000000 ) ) ;
#16363=EDGE_LOOP ( 'NONE', ( #4757, #29647 ) ) ;
#16372=LINE ( 'NONE', #33448, #23148 ) ;
#16439=EDGE_LOOP ( 'NONE', ( #22401, #26965, #10099, #22300 ) ) ;
#16441=CIRCLE ( 'NONE', #26014, 45.00000000000000000 ) ;
#16446=DIRECTION ( 'NONE',  ( -0.000000000000000000, -0.000000000000000000, -1.000000000000000000 ) ) ;
#16505=DIRECTION ( 'NONE',  ( -0.000000000000000000, -0.000000000000000000, -1.000000000000000000 ) ) ;
#16511=CIRCLE ( 'NONE', #3335, 3.500000000000003109 ) ;
#16527=DIRECTION ( 'NONE',  ( -0.000000000000000000, -0.000000000000000000, -1.000000000000000000 ) ) ;
#16546=ORIENTED_EDGE ( 'NONE', *, *, #27912, .T. ) ;
#16629=CARTESIAN_POINT ( 'NONE',  ( 0.000000000000000000, 55.00000000000000000, 5.000000000000000888 ) ) ;
#16682=LINE ( 'NONE', #13854, #13030 ) ;
#16716=EDGE_CURVE ( 'NONE', #25787, #37029, #22095, .T. ) ;
#16738=FACE_BOUND ( 'NONE', #21324, .T. ) ;
#16773=CIRCLE ( 'NONE', #29333, 45.00000000000000711 ) ;
#16778=CIRCLE ( 'NONE', #36535, 3.500000000000003109 ) ;
#16828=EDGE_CURVE ( 'NONE', #5222, #25776, #3959, .T. ) ;
#16878=CARTESIAN_POINT ( 'NONE',  ( -51.13139720814438505, -27.49999999999955591, -5.000000000000000888 ) ) ;
#16905=FACE_BOUND ( 'NONE', #13844, .T. ) ;
#16951=CARTESIAN_POINT ( 'NONE',  ( 51.13139720814400846, -27.50000000000022737, -15.00000000000000000 ) ) ;
#17023=AXIS2_PLACEMENT_3D ( 'NONE', #32995, #13292, #18745 ) ;
#17045=ADVANCED_BREP_SHAPE_REPRESENTATION ( '', ( #20313, #21385 ), #22589 ) ;
#17183=ORIENTED_EDGE ( 'NONE', *, *, #13796, .F. ) ;
#17186=DIRECTION ( 'NONE',  ( 1.000000000000000000, 0.000000000000000000, 0.000000000000000000 ) ) ;
#17219=EDGE_CURVE ( 'NONE', #18518, #6148, #18516, .T. ) ;
#17237=EDGE_LOOP ( 'NONE', ( #3001, #26636, #26143, #35638 ) ) ;
#17302=DIRECTION ( 'NONE',  ( 0.000000000000000000, 0.000000000000000000, 1.000000000000000000 ) ) ;
#17375=CARTESIAN_POINT ( 'NONE',  ( -47.63139720814380951, 27.50000000000055422, -5.000000000000000888 ) ) ;
#17435=ADVANCED_FACE ( 'NONE', ( #25418 ), #19976, .T. ) ;
#17443=CYLINDRICAL_SURFACE ( 'NONE', #4220, 65.00000000000000000 ) ;
#17469=CARTESIAN_POINT ( 'NONE',  ( 0.000000000000000000, 0.000000000000000000, 15.00000000000000000 ) ) ;
#17517=ORIENTED_EDGE ( 'NONE', *, *, #15397, .T. ) ;
#17566=ADVANCED_FACE ( 'NONE', ( #26518 ), #21460, .F. ) ;
#17590=VERTEX_POINT ( 'NONE', #17907 ) ;
#17632=ORIENTED_EDGE ( 'NONE', *, *, #16716, .F. ) ;
#17709=CIRCLE ( 'NONE', #26088, 3.500000000000003109 ) ;
#17716=ORIENTED_EDGE ( 'NONE', *, *, #31504, .F. ) ;
#17724=CARTESIAN_POINT ( 'NONE',  ( 0.000000000000000000, 0.000000000000000000, -5.000000000000000888 ) ) ;
#17787=MECHANICAL_DESIGN_GEOMETRIC_PRESENTATION_REPRESENTATION('',(#413),#1630);
#17802=DIRECTION ( 'NONE',  ( 1.000000000000000000, 0.000000000000000000, 0.000000000000000000 ) ) ;
#17857=PRODUCT_DEFINITION_SHAPE ( 'NONE', 'NONE',  #2674 ) ;
#17907=CARTESIAN_POINT ( 'NONE',  ( -44.13139720814380240, 27.50000000000055422, -5.000000000000000888 ) ) ;
#17910=AXIS2_PLACEMENT_3D ( 'NONE', #30136, #13439, #10450 ) ;
#18023=VERTEX_POINT ( 'NONE', #971 ) ;
#18031=ORIENTED_EDGE ( 'NONE', *, *, #27682, .T. ) ;
#18048=ORIENTED_EDGE ( 'NONE', *, *, #5259, .F. ) ;
#18275=EDGE_LOOP ( 'NONE', ( #25363, #9095 ) ) ;
#18345=CARTESIAN_POINT ( 'NONE',  ( -5.000000000000000000, 24.49489742783178414, -15.00000000000000000 ) ) ;
#18359=VECTOR ( 'NONE', #23701, 1000.000000000000000 ) ;
#18460=CARTESIAN_POINT ( 'NONE',  ( 0.000000000000000000, 0.000000000000000000, 15.00000000000000000 ) ) ;
#18470=CARTESIAN_POINT ( 'NONE',  ( 0.000000000000000000, 55.00000000000000000, -15.00000000000000000 ) ) ;
#18502=CARTESIAN_POINT ( 'NONE',  ( -47.63139720814438505, -27.49999999999955591, 5.000000000000000888 ) ) ;
#18515=DIRECTION ( 'NONE',  ( 1.000000000000000000, 0.000000000000000000, 0.000000000000000000 ) ) ;
#18516=LINE ( 'NONE', #4440, #4617 ) ;
#18517=ADVANCED_FACE ( 'NONE', ( #27716 ), #24739, .T. ) ;
#18518=VERTEX_POINT ( 'NONE', #16127 ) ;
#18542=DIRECTION ( 'NONE',  ( 1.000000000000000000, 0.000000000000000000, 0.000000000000000000 ) ) ;
#18551=DIRECTION ( 'NONE',  ( 1.000000000000000000, 0.000000000000000000, 0.000000000000000000 ) ) ;
#18600=EDGE_LOOP ( 'NONE', ( #9688, #31285 ) ) ;
#18682=AXIS2_PLACEMENT_3D ( 'NONE', #3198, #11454, #36780 ) ;
#18717=FACE_BOUND ( 'NONE', #34869, .T. ) ;
#18719=ORIENTED_EDGE ( 'NONE', *, *, #35780, .F. ) ;
#18745=DIRECTION ( 'NONE',  ( 1.000000000000000000, 0.000000000000000000, 0.000000000000000000 ) ) ;
#18767=( NAMED_UNIT ( * ) PLANE_ANGLE_UNIT ( ) SI_UNIT ( $, .RADIAN. ) );
#18813=ORIENTED_EDGE ( 'NONE', *, *, #679, .F. ) ;
#18840=CARTESIAN_POINT ( 'NONE',  ( -5.000000000000000000, 30.00000000000000355, -15.00000000000000000 ) ) ;
#18890=ORIENTED_EDGE ( 'NONE', *, *, #12405, .F. ) ;
#19065=LINE ( 'NONE', #27838, #2602 ) ;
#19105=CARTESIAN_POINT ( 'NONE',  ( 5.000000000000000000, 30.00000000000000355, -15.00000000000000000 ) ) ;
#19135=DIRECTION ( 'NONE',  ( -0.000000000000000000, -0.000000000000000000, 1.000000000000000000 ) ) ;
#19151=CARTESIAN_POINT ( 'NONE',  ( -65.00000000000000000, 0.000000000000000000, -5.000000000000000000 ) ) ;
#19274=FACE_BOUND ( 'NONE', #29998, .T. ) ;
#19276=AXIS2_PLACEMENT_3D ( 'NONE', #19900, #5846, #14284 ) ;
#19282=CARTESIAN_POINT ( 'NONE',  ( 0.000000000000000000, 0.000000000000000000, 15.00000000000000000 ) ) ;
#19302=EDGE_CURVE ( 'NONE', #23649, #5222, #27207, .T. ) ;
#19324=PRESENTATION_STYLE_ASSIGNMENT (( #23896 ) ) ;
#19347=ORIENTED_EDGE ( 'NONE', *, *, #5259, .T. ) ;
#19372=EDGE_LOOP ( 'NONE', ( #25683, #18890, #30513, #4602 ) ) ;
#19445=AXIS2_PLACEMENT_3D ( 'NONE', #4432, #13238, #30834 ) ;
#19494=EDGE_CURVE ( 'NONE', #37029, #4744, #8630, .T. ) ;
#19533=ORIENTED_EDGE ( 'NONE', *, *, #13268, .F. ) ;
#19539=DIRECTION ( 'NONE',  ( 1.000000000000000000, 0.000000000000000000, 0.000000000000000000 ) ) ;
#19699=VECTOR ( 'NONE', #13947, 1000.000000000000000 ) ;
#19769=EDGE_CURVE ( 'NONE', #5854, #22725, #33191, .T. ) ;
#19811=VERTEX_POINT ( 'NONE', #13469 ) ;
#19835=EDGE_CURVE ( 'NONE', #17590, #22725, #21370, .T. ) ;
#19879=VERTEX_POINT ( 'NONE', #36730 ) ;
#19884=CYLINDRICAL_SURFACE ( 'NONE', #29093, 3.500000000000003109 ) ;
#19900=CARTESIAN_POINT ( 'NONE',  ( 0.000000000000000000, 0.000000000000000000, -5.000000000000000000 ) ) ;
#19906=ORIENTED_EDGE ( 'NONE', *, *, #16716, .T. ) ;
#19908=ORIENTED_EDGE ( 'NONE', *, *, #3281, .F. ) ;
#19945=EDGE_CURVE ( 'NONE', #13995, #1820, #25295, .T. ) ;
#19976=CYLINDRICAL_SURFACE ( 'NONE', #26150, 45.00000000000000000 ) ;
#19990=ADVANCED_FACE ( 'NONE', ( #13052 ), #21855, .F. ) ;
#20003=EDGE_CURVE ( 'NONE', #22186, #1820, #19065, .T. ) ;
#20053=CIRCLE ( 'NONE', #5694, 25.00000000000000000 ) ;
#20064=AXIS2_PLACEMENT_3D ( 'NONE', #23583, #35235, #15141 ) ;
#20102=CIRCLE ( 'NONE', #31464, 3.500000000000000888 ) ;
#20136=DIRECTION ( 'NONE',  ( -0.000000000000000000, 0.000000000000000000, 1.000000000000000000 ) ) ;
#20176=DIRECTION ( 'NONE',  ( 0.000000000000000000, 0.000000000000000000, 1.000000000000000000 ) ) ;
#20287=EDGE_CURVE ( 'NONE', #12924, #13995, #29535, .T. ) ;
#20288=ORIENTED_EDGE ( 'NONE', *, *, #20287, .T. ) ;
#20313=MANIFOLD_SOLID_BREP ( 'CirPattern1', #8219 ) ;
#20370=VECTOR ( 'NONE', #16527, 1000.000000000000000 ) ;
#20426=ORIENTED_EDGE ( 'NONE', *, *, #19945, .F. ) ;
#20443=CARTESIAN_POINT ( 'NONE',  ( -44.13139720814437794, -27.49999999999955591, 5.000000000000000888 ) ) ;
#20567=VECTOR ( 'NONE', #29727, 1000.000000000000000 ) ;
#20598=EDGE_CURVE ( 'NONE', #21193, #18518, #24199, .T. ) ;
#20604=FACE_OUTER_BOUND ( 'NONE', #11257, .T. ) ;
#20627=ORIENTED_EDGE ( 'NONE', *, *, #2368, .F. ) ;
#20629=CARTESIAN_POINT ( 'NONE',  ( 0.000000000000000000, -55.00000000000000000, -5.000000000000000888 ) ) ;
#20633=ORIENTED_EDGE ( 'NONE', *, *, #6588, .T. ) ;
#20658=EDGE_CURVE ( 'NONE', #3324, #14961, #9595, .T. ) ;
#20687=APPLICATION_CONTEXT ( 'automotive_design' ) ;
#20690=ADVANCED_FACE ( 'NONE', ( #21756 ), #15767, .F. ) ;
#20703=DIRECTION ( 'NONE',  ( -0.000000000000000000, -0.000000000000000000, 1.000000000000000000 ) ) ;
#20729=AXIS2_PLACEMENT_3D ( 'NONE', #33555, #16120, #24916 ) ;
#20813=EDGE_LOOP ( 'NONE', ( #24549, #25831, #26491, #9008 ) ) ;
#20816=AXIS2_PLACEMENT_3D ( 'NONE', #25405, #34233, #7971 ) ;
#20902=CARTESIAN_POINT ( 'NONE',  ( -65.00000000000000000, 0.000000000000000000, 5.000000000000000000 ) ) ;
#20936=DIRECTION ( 'NONE',  ( 1.000000000000000000, 0.000000000000000000, -0.000000000000000000 ) ) ;
#20938=VERTEX_POINT ( 'NONE', #16878 ) ;
#20963=EDGE_CURVE ( 'NONE', #14395, #3448, #21844, .T. ) ;
#20966=DIRECTION ( 'NONE',  ( 0.000000000000000000, 0.000000000000000000, 1.000000000000000000 ) ) ;
#21037=DIRECTION ( 'NONE',  ( 0.000000000000000000, 0.000000000000000000, 1.000000000000000000 ) ) ;
#21193=VERTEX_POINT ( 'NONE', #16111 ) ;
#21315=VERTEX_POINT ( 'NONE', #28261 ) ;
#21324=EDGE_LOOP ( 'NONE', ( #7246, #33580 ) ) ;
#21370=LINE ( 'NONE', #36372, #36202 ) ;
#21385=AXIS2_PLACEMENT_3D ( 'NONE', #8896, #30384, #36396 ) ;
#21388=CARTESIAN_POINT ( 'NONE',  ( 0.000000000000000000, 0.000000000000000000, -15.00000000000000000 ) ) ;
#21460=CYLINDRICAL_SURFACE ( 'NONE', #36363, 3.500000000000000888 ) ;
#21484=AXIS2_PLACEMENT_3D ( 'NONE', #21955, #16505, #14254 ) ;
#21521=AXIS2_PLACEMENT_3D ( 'NONE', #35978, #2202, #2009 ) ;
#21574=ORIENTED_EDGE ( 'NONE', *, *, #33249, .F. ) ;
#21595=CARTESIAN_POINT ( 'NONE',  ( 0.000000000000000000, -55.00000000000000000, -15.00000000000000000 ) ) ;
#21756=FACE_OUTER_BOUND ( 'NONE', #17237, .T. ) ;
#21759=EDGE_LOOP ( 'NONE', ( #30312, #1187, #36169, #8642 ) ) ;
#21844=CIRCLE ( 'NONE', #26013, 3.500000000000003109 ) ;
#21855=CYLINDRICAL_SURFACE ( 'NONE', #19445, 3.500000000000003109 ) ;
#21868=ORIENTED_EDGE ( 'NONE', *, *, #3160, .F. ) ;
#21955=CARTESIAN_POINT ( 'NONE',  ( 0.000000000000000000, 0.000000000000000000, 15.00000000000000000 ) ) ;
#21982=DIRECTION ( 'NONE',  ( -0.000000000000000000, -0.000000000000000000, -1.000000000000000000 ) ) ;
#21983=CYLINDRICAL_SURFACE ( 'NONE', #27464, 3.500000000000003109 ) ;
#22051=ADVANCED_FACE ( 'NONE', ( #35357 ), #4383, .F. ) ;
#22066=ORIENTED_EDGE ( 'NONE', *, *, #20658, .T. ) ;
#22091=ADVANCED_FACE ( 'NONE', ( #6813 ), #29680, .T. ) ;
#22095=CIRCLE ( 'NONE', #4133, 65.00000000000000000 ) ;
#22159=FACE_OUTER_BOUND ( 'NONE', #33357, .T. ) ;
#22180=CIRCLE ( 'NONE', #12574, 45.00000000000000711 ) ;
#22181=CARTESIAN_POINT ( 'NONE',  ( 51.13139720814419320, 27.49999999999988987, -5.000000000000000888 ) ) ;
#22186=VERTEX_POINT ( 'NONE', #7764 ) ;
#22300=ORIENTED_EDGE ( 'NONE', *, *, #35780, .T. ) ;
#22303=CIRCLE ( 'NONE', #27695, 3.500000000000003109 ) ;
#22345=CARTESIAN_POINT ( 'NONE',  ( 47.63139720814400846, -27.50000000000022737, -15.00000000000000000 ) ) ;
#22401=ORIENTED_EDGE ( 'NONE', *, *, #27682, .F. ) ;
#22462=CARTESIAN_POINT ( 'NONE',  ( -25.00000000000000000, 0.000000000000000000, -15.00000000000000000 ) ) ;
#22488=CARTESIAN_POINT ( 'NONE',  ( -45.00000000000000000, 0.000000000000000000, -5.000000000000000888 ) ) ;
#22548=ORIENTED_EDGE ( 'NONE', *, *, #31325, .T. ) ;
#22589=( GEOMETRIC_REPRESENTATION_CONTEXT ( 3 ) GLOBAL_UNCERTAINTY_ASSIGNED_CONTEXT ( ( #7321 ) ) GLOBAL_UNIT_ASSIGNED_CONTEXT ( ( #5910, #14694, #31572 ) ) REPRESENTATION_CONTEXT ( 'NONE', 'WORKASPACE' ) );
#22641=AXIS2_PLACEMENT_3D ( 'NONE', #17375, #28795, #2947 ) ;
#22684=DIRECTION ( 'NONE',  ( 1.000000000000000000, 0.000000000000000000, 0.000000000000000000 ) ) ;
#22725=VERTEX_POINT ( 'NONE', #26751 ) ;
#22732=CARTESIAN_POINT ( 'NONE',  ( -3.500000000000000888, 55.00000000000000000, -5.000000000000000888 ) ) ;
#22821=LINE ( 'NONE', #14374, #27425 ) ;
#22878=ADVANCED_FACE ( 'NONE', ( #27112 ), #7071, .F. ) ;
#22907=DIRECTION ( 'NONE',  ( 1.000000000000000000, 0.000000000000000000, 0.000000000000000000 ) ) ;
#22950=DIRECTION ( 'NONE',  ( -0.000000000000000000, -0.000000000000000000, -1.000000000000000000 ) ) ;
#22964=AXIS2_PLACEMENT_3D ( 'NONE', #33832, #30642, #25393 ) ;
#23033=CARTESIAN_POINT ( 'NONE',  ( 0.000000000000000000, -55.00000000000000000, 5.000000000000000888 ) ) ;
#23120=DIRECTION ( 'NONE',  ( 0.000000000000000000, 0.000000000000000000, 1.000000000000000000 ) ) ;
#23148=VECTOR ( 'NONE', #13551, 1000.000000000000000 ) ;
#23149=VECTOR ( 'NONE', #28056, 1000.000000000000000 ) ;
#23334=ORIENTED_EDGE ( 'NONE', *, *, #20963, .F. ) ;
#23422=AXIS2_PLACEMENT_3D ( 'NONE', #29948, #35586, #32953 ) ;
#23543=CARTESIAN_POINT ( 'NONE',  ( -51.13139720814380951, 27.50000000000055422, -15.00000000000000000 ) ) ;
#23544=DIRECTION ( 'NONE',  ( 1.000000000000000000, 0.000000000000000000, 0.000000000000000000 ) ) ;
#23570=VECTOR ( 'NONE', #36430, 1000.000000000000000 ) ;
#23583=CARTESIAN_POINT ( 'NONE',  ( 0.000000000000000000, 55.00000000000000000, -5.000000000000000888 ) ) ;
#23596=AXIS2_PLACEMENT_3D ( 'NONE', #17724, #20176, #26532 ) ;
#23629=CARTESIAN_POINT ( 'NONE',  ( 45.00000000000000000, 5.510910596163089556E-15, 15.00000000000000000 ) ) ;
#23647=CARTESIAN_POINT ( 'NONE',  ( -3.500000000000000888, 55.00000000000000000, -15.00000000000000000 ) ) ;
#23649=VERTEX_POINT ( 'NONE', #3067 ) ;
#23701=DIRECTION ( 'NONE',  ( -0.000000000000000000, 1.000000000000000000, 0.000000000000000000 ) ) ;
#23750=CARTESIAN_POINT ( 'NONE',  ( 5.000000000000000000, 25.00000000000000000, -15.00000000000000000 ) ) ;
#23781=CARTESIAN_POINT ( 'NONE',  ( 0.000000000000000000, 55.00000000000000000, 5.000000000000000888 ) ) ;
#23896=SURFACE_STYLE_USAGE ( .BOTH. , #10705 ) ;
#23909=CARTESIAN_POINT ( 'NONE',  ( 51.13139720814419320, 27.49999999999988987, 5.000000000000000888 ) ) ;
#24024=DIRECTION ( 'NONE',  ( 1.000000000000000000, 0.000000000000000000, 0.000000000000000000 ) ) ;
#24061=CIRCLE ( 'NONE', #18682, 3.500000000000003109 ) ;
#24119=FILL_AREA_STYLE_COLOUR ( '', #6795 ) ;
#24154=CARTESIAN_POINT ( 'NONE',  ( 0.000000000000000000, 0.000000000000000000, -5.000000000000000888 ) ) ;
#24199=CIRCLE ( 'NONE', #8033, 3.500000000000000888 ) ;
#24224=ORIENTED_EDGE ( 'NONE', *, *, #10619, .F. ) ;
#24243=DIRECTION ( 'NONE',  ( 1.000000000000000000, 0.000000000000000000, 0.000000000000000000 ) ) ;
#24251=AXIS2_PLACEMENT_3D ( 'NONE', #19282, #24905, #24719 ) ;
#24282=CARTESIAN_POINT ( 'NONE',  ( 0.000000000000000000, 0.000000000000000000, -5.000000000000000000 ) ) ;
#24329=AXIS2_PLACEMENT_3D ( 'NONE', #9836, #35924, #7407 ) ;
#24335=VERTEX_POINT ( 'NONE', #31623 ) ;
#24370=VERTEX_POINT ( 'NONE', #5761 ) ;
#24426=CARTESIAN_POINT ( 'NONE',  ( -47.63139720814380951, 27.50000000000055422, 5.000000000000000888 ) ) ;
#24484=FACE_OUTER_BOUND ( 'NONE', #1420, .T. ) ;
#24485=LINE ( 'NONE', #3673, #2891 ) ;
#24489=DIRECTION ( 'NONE',  ( 0.000000000000000000, 0.000000000000000000, 1.000000000000000000 ) ) ;
#24525=CIRCLE ( 'NONE', #13727, 65.00000000000000000 ) ;
#24549=ORIENTED_EDGE ( 'NONE', *, *, #8044, .F. ) ;
#24587=CIRCLE ( 'NONE', #5416, 3.500000000000000888 ) ;
#24629=VERTEX_POINT ( 'NONE', #36072 ) ;
#24631=DIRECTION ( 'NONE',  ( 0.000000000000000000, 0.000000000000000000, 1.000000000000000000 ) ) ;
#24648=DIRECTION ( 'NONE',  ( 0.000000000000000000, 0.000000000000000000, 1.000000000000000000 ) ) ;
#24714=EDGE_LOOP ( 'NONE', ( #34486, #3037, #34943, #35511 ) ) ;
#24719=DIRECTION ( 'NONE',  ( 1.000000000000000000, 0.000000000000000000, 0.000000000000000000 ) ) ;
#24739=CYLINDRICAL_SURFACE ( 'NONE', #9128, 65.00000000000000000 ) ;
#24746=DIRECTION ( 'NONE',  ( 0.000000000000000000, 0.000000000000000000, 1.000000000000000000 ) ) ;
#24774=ORIENTED_EDGE ( 'NONE', *, *, #33875, .T. ) ;
#24838=EDGE_LOOP ( 'NONE', ( #17183, #1009 ) ) ;
#24905=DIRECTION ( 'NONE',  ( 0.000000000000000000, 0.000000000000000000, 1.000000000000000000 ) ) ;
#24916=DIRECTION ( 'NONE',  ( 1.000000000000000000, 0.000000000000000000, 0.000000000000000000 ) ) ;
#25072=CARTESIAN_POINT ( 'NONE',  ( 0.000000000000000000, 0.000000000000000000, 15.00000000000000000 ) ) ;
#25211=CYLINDRICAL_SURFACE ( 'NONE', #14114, 45.00000000000000000 ) ;
#25295=LINE ( 'NONE', #28456, #25437 ) ;
#25363=ORIENTED_EDGE ( 'NONE', *, *, #8739, .F. ) ;
#25391=VECTOR ( 'NONE', #1909, 1000.000000000000000 ) ;
#25393=DIRECTION ( 'NONE',  ( 1.000000000000000000, 0.000000000000000000, 0.000000000000000000 ) ) ;
#25405=CARTESIAN_POINT ( 'NONE',  ( 47.63139720814418610, 27.49999999999988987, -5.000000000000000888 ) ) ;
#25418=FACE_OUTER_BOUND ( 'NONE', #2096, .T. ) ;
#25427=VERTEX_POINT ( 'NONE', #3692 ) ;
#25431=LINE ( 'NONE', #5392, #27367 ) ;
#25437=VECTOR ( 'NONE', #5592, 1000.000000000000000 ) ;
#25534=VERTEX_POINT ( 'NONE', #1425 ) ;
#25588=LINE ( 'NONE', #34771, #524 ) ;
#25604=EDGE_LOOP ( 'NONE', ( #22548, #216, #16546, #20288, #18813, #18048 ) ) ;
#25683=ORIENTED_EDGE ( 'NONE', *, *, #27190, .F. ) ;
#25698=DIRECTION ( 'NONE',  ( 0.000000000000000000, 0.000000000000000000, 1.000000000000000000 ) ) ;
#25749=CIRCLE ( 'NONE', #35338, 25.00000000000000000 ) ;
#25764=AXIS2_PLACEMENT_3D ( 'NONE', #31563, #20136, #2150 ) ;
#25776=VERTEX_POINT ( 'NONE', #23909 ) ;
#25787=VERTEX_POINT ( 'NONE', #6092 ) ;
#25831=ORIENTED_EDGE ( 'NONE', *, *, #12384, .T. ) ;
#25857=DIRECTION ( 'NONE',  ( -0.000000000000000000, -0.000000000000000000, 1.000000000000000000 ) ) ;
#26013=AXIS2_PLACEMENT_3D ( 'NONE', #14251, #25698, #6412 ) ;
#26014=AXIS2_PLACEMENT_3D ( 'NONE', #24154, #3725, #18551 ) ;
#26015=DIRECTION ( 'NONE',  ( 0.000000000000000000, 0.000000000000000000, 1.000000000000000000 ) ) ;
#26088=AXIS2_PLACEMENT_3D ( 'NONE', #37076, #674, #23544 ) ;
#26143=ORIENTED_EDGE ( 'NONE', *, *, #1750, .T. ) ;
#26150=AXIS2_PLACEMENT_3D ( 'NONE', #5730, #8913, #31932 ) ;
#26188=DIRECTION ( 'NONE',  ( 0.000000000000000000, 0.000000000000000000, 1.000000000000000000 ) ) ;
#26190=EDGE_CURVE ( 'NONE', #30372, #30464, #31884, .T. ) ;
#26255=DIRECTION ( 'NONE',  ( 0.000000000000000000, 0.000000000000000000, 1.000000000000000000 ) ) ;
#26491=ORIENTED_EDGE ( 'NONE', *, *, #33875, .F. ) ;
#26509=DIRECTION ( 'NONE',  ( -1.000000000000000000, 0.000000000000000000, 0.000000000000000000 ) ) ;
#26518=FACE_OUTER_BOUND ( 'NONE', #21759, .T. ) ;
#26532=DIRECTION ( 'NONE',  ( 1.000000000000000000, 0.000000000000000000, 0.000000000000000000 ) ) ;
#26546=( NAMED_UNIT ( * ) PLANE_ANGLE_UNIT ( ) SI_UNIT ( $, .RADIAN. ) );
#26574=STYLED_ITEM ( 'NONE', ( #1419 ), #20313 ) ;
#26610=DIRECTION ( 'NONE',  ( 1.000000000000000000, 0.000000000000000000, 0.000000000000000000 ) ) ;
#26613=VECTOR ( 'NONE', #7528, 1000.000000000000000 ) ;
#26636=ORIENTED_EDGE ( 'NONE', *, *, #27190, .T. ) ;
#26751=CARTESIAN_POINT ( 'NONE',  ( -44.13139720814380240, 27.50000000000055422, 5.000000000000000888 ) ) ;
#26804=ORIENTED_EDGE ( 'NONE', *, *, #8537, .T. ) ;
#26861=VERTEX_POINT ( 'NONE', #8722 ) ;
#26891=CARTESIAN_POINT ( 'NONE',  ( 44.13139720814418610, 27.49999999999988987, 5.000000000000000888 ) ) ;
#26929=FILL_AREA_STYLE ('',( #24119 ) ) ;
#26965=ORIENTED_EDGE ( 'NONE', *, *, #6588, .F. ) ;
#27020=ADVANCED_FACE ( 'NONE', ( #35372 ), #31935, .F. ) ;
#27084=CIRCLE ( 'NONE', #34882, 25.00000000000000000 ) ;
#27089=DIRECTION ( 'NONE',  ( -0.000000000000000000, 1.000000000000000000, 0.000000000000000000 ) ) ;
#27112=FACE_OUTER_BOUND ( 'NONE', #29249, .T. ) ;
#27178=ORIENTED_EDGE ( 'NONE', *, *, #19769, .F. ) ;
#27190=EDGE_CURVE ( 'NONE', #21193, #19879, #4226, .T. ) ;
#27192=ORIENTED_EDGE ( 'NONE', *, *, #4561, .F. ) ;
#27207=LINE ( 'NONE', #33777, #25391 ) ;
#27218=LINE ( 'NONE', #30419, #28356 ) ;
#27327=ORIENTED_EDGE ( 'NONE', *, *, #11189, .T. ) ;
#27332=CIRCLE ( 'NONE', #11741, 3.500000000000003109 ) ;
#27365=CARTESIAN_POINT ( 'NONE',  ( -47.63139720814438505, -27.49999999999955591, -15.00000000000000000 ) ) ;
#27367=VECTOR ( 'NONE', #17186, 1000.000000000000000 ) ;
#27394=LINE ( 'NONE', #29628, #4084 ) ;
#27425=VECTOR ( 'NONE', #14544, 1000.000000000000000 ) ;
#27436=CARTESIAN_POINT ( 'NONE',  ( 47.63139720814418610, 27.49999999999988987, -15.00000000000000000 ) ) ;
#27464=AXIS2_PLACEMENT_3D ( 'NONE', #22345, #8098, #19539 ) ;
#27519=AXIS2_PLACEMENT_3D ( 'NONE', #9111, #35196, #20936 ) ;
#27524=FACE_BOUND ( 'NONE', #24838, .T. ) ;
#27563=CYLINDRICAL_SURFACE ( 'NONE', #13079, 3.500000000000003109 ) ;
#27597=LINE ( 'NONE', #33206, #26613 ) ;
#27682=EDGE_CURVE ( 'NONE', #14395, #24629, #27597, .T. ) ;
#27685=CARTESIAN_POINT ( 'NONE',  ( -47.63139720814438505, -27.49999999999955591, 5.000000000000000888 ) ) ;
#27695=AXIS2_PLACEMENT_3D ( 'NONE', #32867, #13340, #6986 ) ;
#27715=ORIENTED_EDGE ( 'NONE', *, *, #5291, .F. ) ;
#27716=FACE_OUTER_BOUND ( 'NONE', #34684, .T. ) ;
#27722=FACE_OUTER_BOUND ( 'NONE', #1002, .T. ) ;
#27825=EDGE_LOOP ( 'NONE', ( #35631, #30940, #32662, #14451 ) ) ;
#27838=CARTESIAN_POINT ( 'NONE',  ( 5.000000000000000000, 25.00000000000000000, 15.00000000000000000 ) ) ;
#27875=FACE_BOUND ( 'NONE', #30421, .T. ) ;
#27882=DIRECTION ( 'NONE',  ( 1.000000000000000000, 0.000000000000000000, 0.000000000000000000 ) ) ;
#27899=ORIENTED_EDGE ( 'NONE', *, *, #3281, .T. ) ;
#27907=AXIS2_PLACEMENT_3D ( 'NONE', #21388, #29822, #24024 ) ;
#27912=EDGE_CURVE ( 'NONE', #26861, #12924, #34419, .T. ) ;
#28018=AXIS2_PLACEMENT_3D ( 'NONE', #1817, #12674, #18515 ) ;
#28056=DIRECTION ( 'NONE',  ( -0.000000000000000000, -0.000000000000000000, 1.000000000000000000 ) ) ;
#28096=ORIENTED_EDGE ( 'NONE', *, *, #11129, .F. ) ;
#28131=AXIS2_PLACEMENT_3D ( 'NONE', #3854, #26188, #9504 ) ;
#28139=ORIENTED_EDGE ( 'NONE', *, *, #679, .T. ) ;
#28158=EDGE_CURVE ( 'NONE', #29596, #26861, #20053, .T. ) ;
#28188=FACE_OUTER_BOUND ( 'NONE', #24714, .T. ) ;
#28261=CARTESIAN_POINT ( 'NONE',  ( 25.00000000000000000, 3.061616997868383043E-15, 15.00000000000000000 ) ) ;
#28317=CARTESIAN_POINT ( 'NONE',  ( 65.00000000000000000, 7.960204194457797252E-15, 5.000000000000000000 ) ) ;
#28356=VECTOR ( 'NONE', #21982, 1000.000000000000000 ) ;
#28386=CARTESIAN_POINT ( 'NONE',  ( 65.00000000000000000, 7.960204194457797252E-15, 5.000000000000000000 ) ) ;
#28456=CARTESIAN_POINT ( 'NONE',  ( 5.000000000000000000, 30.00000000000000355, -15.00000000000000000 ) ) ;
#28468=CARTESIAN_POINT ( 'NONE',  ( -45.00000000000000000, 0.000000000000000000, 15.00000000000000000 ) ) ;
#28476=ORIENTED_EDGE ( 'NONE', *, *, #4185, .T. ) ;
#28490=CIRCLE ( 'NONE', #12306, 3.500000000000003109 ) ;
#28699=CARTESIAN_POINT ( 'NONE',  ( 0.000000000000000000, 0.000000000000000000, 5.000000000000000000 ) ) ;
#28795=DIRECTION ( 'NONE',  ( 0.000000000000000000, 0.000000000000000000, 1.000000000000000000 ) ) ;
#28835=EDGE_LOOP ( 'NONE', ( #36184, #31316 ) ) ;
#28849=ADVANCED_FACE ( 'NONE', ( #28188 ), #25211, .T. ) ;
#28882=EDGE_LOOP ( 'NONE', ( #13017, #13358 ) ) ;
#28885=DIRECTION ( 'NONE',  ( 1.000000000000000000, 0.000000000000000000, 0.000000000000000000 ) ) ;
#28913=DIRECTION ( 'NONE',  ( 1.000000000000000000, 0.000000000000000000, 0.000000000000000000 ) ) ;
#28943=CIRCLE ( 'NONE', #13396, 25.00000000000000000 ) ;
#28984=CARTESIAN_POINT ( 'NONE',  ( -51.13139720814380951, 27.50000000000055422, 5.000000000000000888 ) ) ;
#29085=DIRECTION ( 'NONE',  ( -0.000000000000000000, -0.000000000000000000, -1.000000000000000000 ) ) ;
#29093=AXIS2_PLACEMENT_3D ( 'NONE', #30947, #36766, #11441 ) ;
#29121=DIRECTION ( 'NONE',  ( 1.000000000000000000, 0.000000000000000000, 0.000000000000000000 ) ) ;
#29126=CARTESIAN_POINT ( 'NONE',  ( 45.00000000000000000, 5.510910596163089556E-15, -5.000000000000000888 ) ) ;
#29130=PRODUCT_DEFINITION_FORMATION_WITH_SPECIFIED_SOURCE ( 'ANY', '', #10399, .NOT_KNOWN. ) ;
#29249=EDGE_LOOP ( 'NONE', ( #12657, #27327, #14256, #21868 ) ) ;
#29252=ADVANCED_FACE ( 'NONE', ( #22159 ), #19884, .F. ) ;
#29272=CIRCLE ( 'NONE', #7159, 65.00000000000000000 ) ;
#29333=AXIS2_PLACEMENT_3D ( 'NONE', #35317, #21037, #1174 ) ;
#29410=CARTESIAN_POINT ( 'NONE',  ( -45.00000000000000711, 0.000000000000000000, 5.000000000000000000 ) ) ;
#29415=EDGE_LOOP ( 'NONE', ( #20627, #14189, #2296, #32555 ) ) ;
#29535=LINE ( 'NONE', #23750, #20567 ) ;
#29596=VERTEX_POINT ( 'NONE', #22462 ) ;
#29628=CARTESIAN_POINT ( 'NONE',  ( 51.13139720814419320, 27.49999999999988987, -15.00000000000000000 ) ) ;
#29634=AXIS2_PLACEMENT_3D ( 'NONE', #23781, #20966, #3717 ) ;
#29647=ORIENTED_EDGE ( 'NONE', *, *, #31504, .T. ) ;
#29680=CYLINDRICAL_SURFACE ( 'NONE', #30037, 45.00000000000000000 ) ;
#29727=DIRECTION ( 'NONE',  ( -0.000000000000000000, 1.000000000000000000, 0.000000000000000000 ) ) ;
#29822=DIRECTION ( 'NONE',  ( 0.000000000000000000, 0.000000000000000000, 1.000000000000000000 ) ) ;
#29863=DIRECTION ( 'NONE',  ( 1.000000000000000000, 0.000000000000000000, 0.000000000000000000 ) ) ;
#29948=CARTESIAN_POINT ( 'NONE',  ( -5.000000000000000000, 25.00000000000000000, -15.00000000000000000 ) ) ;
#29963=EDGE_LOOP ( 'NONE', ( #31677, #11254 ) ) ;
#29998=EDGE_LOOP ( 'NONE', ( #21574, #27178 ) ) ;
#30009=EDGE_LOOP ( 'NONE', ( #15231, #8924 ) ) ;
#30017=ORIENTED_EDGE ( 'NONE', *, *, #11189, .F. ) ;
#30019=ADVANCED_FACE ( 'NONE', ( #35916 ), #10222, .T. ) ;
#30037=AXIS2_PLACEMENT_3D ( 'NONE', #18460, #30239, #26509 ) ;
#30054=DIRECTION ( 'NONE',  ( -0.000000000000000000, -0.000000000000000000, 1.000000000000000000 ) ) ;
#30131=FACE_BOUND ( 'NONE', #35724, .T. ) ;
#30136=CARTESIAN_POINT ( 'NONE',  ( 0.000000000000000000, 0.000000000000000000, 15.00000000000000000 ) ) ;
#30211=ORIENTED_EDGE ( 'NONE', *, *, #19302, .T. ) ;
#30239=DIRECTION ( 'NONE',  ( -0.000000000000000000, -0.000000000000000000, -1.000000000000000000 ) ) ;
#30251=DIRECTION ( 'NONE',  ( -0.000000000000000000, -0.000000000000000000, 1.000000000000000000 ) ) ;
#30256=DIRECTION ( 'NONE',  ( 0.000000000000000000, -1.000000000000000000, 0.000000000000000000 ) ) ;
#30312=ORIENTED_EDGE ( 'NONE', *, *, #20658, .F. ) ;
#30372=VERTEX_POINT ( 'NONE', #29126 ) ;
#30384=DIRECTION ( 'NONE',  ( 0.000000000000000000, 0.000000000000000000, 1.000000000000000000 ) ) ;
#30419=CARTESIAN_POINT ( 'NONE',  ( -25.00000000000000000, 0.000000000000000000, 15.00000000000000000 ) ) ;
#30421=EDGE_LOOP ( 'NONE', ( #27192, #34224 ) ) ;
#30428=CIRCLE ( 'NONE', #8880, 45.00000000000000000 ) ;
#30464=VERTEX_POINT ( 'NONE', #30598 ) ;
#30474=CARTESIAN_POINT ( 'NONE',  ( -44.13139720814437794, -27.49999999999955591, -5.000000000000000888 ) ) ;
#30500=EDGE_CURVE ( 'NONE', #31944, #25427, #30428, .T. ) ;
#30513=ORIENTED_EDGE ( 'NONE', *, *, #17219, .T. ) ;
#30529=FACE_BOUND ( 'NONE', #209, .T. ) ;
#30540=ORIENTED_EDGE ( 'NONE', *, *, #33249, .T. ) ;
#30598=CARTESIAN_POINT ( 'NONE',  ( 45.00000000000000000, 5.510910596163089556E-15, -15.00000000000000000 ) ) ;
#30604=DIRECTION ( 'NONE',  ( 0.000000000000000000, 0.000000000000000000, 1.000000000000000000 ) ) ;
#30642=DIRECTION ( 'NONE',  ( 0.000000000000000000, 0.000000000000000000, 1.000000000000000000 ) ) ;
#30690=FACE_OUTER_BOUND ( 'NONE', #13478, .T. ) ;
#30742=( LENGTH_UNIT ( ) NAMED_UNIT ( * ) SI_UNIT ( .MILLI., .METRE. ) );
#30745=VECTOR ( 'NONE', #36382, 1000.000000000000000 ) ;
#30785=ADVANCED_FACE ( 'NONE', ( #27722 ), #27563, .F. ) ;
#30834=DIRECTION ( 'NONE',  ( 1.000000000000000000, 0.000000000000000000, 0.000000000000000000 ) ) ;
#30940=ORIENTED_EDGE ( 'NONE', *, *, #15517, .F. ) ;
#30947=CARTESIAN_POINT ( 'NONE',  ( -47.63139720814380951, 27.50000000000055422, -15.00000000000000000 ) ) ;
#30953=AXIS2_PLACEMENT_3D ( 'NONE', #18840, #30256, #3241 ) ;
#30965=ORIENTED_EDGE ( 'NONE', *, *, #2557, .T. ) ;
#31009=ORIENTED_EDGE ( 'NONE', *, *, #36027, .F. ) ;
#31149=LINE ( 'NONE', #5086, #20370 ) ;
#31281=LINE ( 'NONE', #28468, #30745 ) ;
#31285=ORIENTED_EDGE ( 'NONE', *, *, #3882, .F. ) ;
#31316=ORIENTED_EDGE ( 'NONE', *, *, #6873, .F. ) ;
#31325=EDGE_CURVE ( 'NONE', #10522, #29596, #28943, .T. ) ;
#31364=ORIENTED_EDGE ( 'NONE', *, *, #34520, .F. ) ;
#31447=ORIENTED_EDGE ( 'NONE', *, *, #10619, .T. ) ;
#31464=AXIS2_PLACEMENT_3D ( 'NONE', #16629, #7830, #7994 ) ;
#31504=EDGE_CURVE ( 'NONE', #30372, #14697, #2051, .T. ) ;
#31523=DIRECTION ( 'NONE',  ( 0.000000000000000000, -0.000000000000000000, 1.000000000000000000 ) ) ;
#31538=DIRECTION ( 'NONE',  ( -0.000000000000000000, -0.000000000000000000, -1.000000000000000000 ) ) ;
#31563=CARTESIAN_POINT ( 'NONE',  ( 47.63139720814400846, -27.50000000000022737, -15.00000000000000000 ) ) ;
#31572=( NAMED_UNIT ( * ) SI_UNIT ( $, .STERADIAN. ) SOLID_ANGLE_UNIT ( ) );
#31623=CARTESIAN_POINT ( 'NONE',  ( 3.500000000000000888, 55.00000000000000000, -5.000000000000000888 ) ) ;
#31677=ORIENTED_EDGE ( 'NONE', *, *, #15517, .T. ) ;
#31822=VERTEX_POINT ( 'NONE', #11618 ) ;
#31884=LINE ( 'NONE', #15038, #4002 ) ;
#31898=CARTESIAN_POINT ( 'NONE',  ( 5.000000000000000000, 30.00000000000000355, 15.00000000000000000 ) ) ;
#31916=ORIENTED_EDGE ( 'NONE', *, *, #20003, .F. ) ;
#31932=DIRECTION ( 'NONE',  ( -1.000000000000000000, 0.000000000000000000, 0.000000000000000000 ) ) ;
#31935=CYLINDRICAL_SURFACE ( 'NONE', #8104, 3.500000000000000888 ) ;
#31944=VERTEX_POINT ( 'NONE', #23629 ) ;
#32145=FACE_OUTER_BOUND ( 'NONE', #15963, .T. ) ;
#32272=EDGE_LOOP ( 'NONE', ( #19533, #22066, #3769, #36506 ) ) ;
#32301=EDGE_CURVE ( 'NONE', #14961, #13777, #36827, .T. ) ;
#32304=EDGE_CURVE ( 'NONE', #24335, #3324, #4500, .T. ) ;
#32449=DIRECTION ( 'NONE',  ( 0.000000000000000000, 0.000000000000000000, 1.000000000000000000 ) ) ;
#32555=ORIENTED_EDGE ( 'NONE', *, *, #19835, .F. ) ;
#32622=CIRCLE ( 'NONE', #24251, 45.00000000000000000 ) ;
#32662=ORIENTED_EDGE ( 'NONE', *, *, #11289, .T. ) ;
#32686=DIRECTION ( 'NONE',  ( -0.000000000000000000, -0.000000000000000000, -1.000000000000000000 ) ) ;
#32743=CARTESIAN_POINT ( 'NONE',  ( 3.500000000000000888, -55.00000000000000000, 5.000000000000000888 ) ) ;
#32758=AXIS2_PLACEMENT_3D ( 'NONE', #27685, #33695, #13072 ) ;
#32774=CYLINDRICAL_SURFACE ( 'NONE', #7773, 3.500000000000003109 ) ;
#32806=ORIENTED_EDGE ( 'NONE', *, *, #35183, .F. ) ;
#32867=CARTESIAN_POINT ( 'NONE',  ( -47.63139720814438505, -27.49999999999955591, -5.000000000000000888 ) ) ;
#32878=ORIENTED_EDGE ( 'NONE', *, *, #3882, .T. ) ;
#32916=DIRECTION ( 'NONE',  ( -0.000000000000000000, -0.000000000000000000, 1.000000000000000000 ) ) ;
#32924=CARTESIAN_POINT ( 'NONE',  ( 44.13139720814400135, -27.50000000000022737, -5.000000000000000888 ) ) ;
#32953=DIRECTION ( 'NONE',  ( 0.000000000000000000, 0.000000000000000000, -1.000000000000000000 ) ) ;
#32993=CARTESIAN_POINT ( 'NONE',  ( 0.000000000000000000, 0.000000000000000000, -15.00000000000000000 ) ) ;
#32995=CARTESIAN_POINT ( 'NONE',  ( -47.63139720814380951, 27.50000000000055422, 5.000000000000000888 ) ) ;
#33167=DIRECTION ( 'NONE',  ( 1.000000000000000000, 0.000000000000000000, 0.000000000000000000 ) ) ;
#33191=CIRCLE ( 'NONE', #17023, 3.500000000000003109 ) ;
#33193=ORIENTED_EDGE ( 'NONE', *, *, #3696, .F. ) ;
#33206=CARTESIAN_POINT ( 'NONE',  ( 44.13139720814400135, -27.50000000000022737, -15.00000000000000000 ) ) ;
#33221=LINE ( 'NONE', #13174, #23570 ) ;
#33228=DIRECTION ( 'NONE',  ( 1.000000000000000000, 0.000000000000000000, 0.000000000000000000 ) ) ;
#33249=EDGE_CURVE ( 'NONE', #22725, #5854, #12336, .T. ) ;
#33275=PLANE ( 'NONE',  #24329 ) ;
#33357=EDGE_LOOP ( 'NONE', ( #33193, #19908, #13216, #30540 ) ) ;
#33395=DIRECTION ( 'NONE',  ( -0.000000000000000000, -0.000000000000000000, 1.000000000000000000 ) ) ;
#33448=CARTESIAN_POINT ( 'NONE',  ( 45.00000000000000000, 5.510910596163089556E-15, 15.00000000000000000 ) ) ;
#33474=SHAPE_REPRESENTATION ( 'rotor hub', ( #21385 ), #22589 ) ;
#33505=DIRECTION ( 'NONE',  ( 0.000000000000000000, 0.000000000000000000, 1.000000000000000000 ) ) ;
#33555=CARTESIAN_POINT ( 'NONE',  ( 47.63139720814418610, 27.49999999999988987, 5.000000000000000888 ) ) ;
#33580=ORIENTED_EDGE ( 'NONE', *, *, #9585, .T. ) ;
#33695=DIRECTION ( 'NONE',  ( 0.000000000000000000, 0.000000000000000000, 1.000000000000000000 ) ) ;
#33760=FACE_OUTER_BOUND ( 'NONE', #20813, .T. ) ;
#33777=CARTESIAN_POINT ( 'NONE',  ( 44.13139720814418610, 27.49999999999988987, -15.00000000000000000 ) ) ;
#33793=VECTOR ( 'NONE', #2639, 1000.000000000000000 ) ;
#33832=CARTESIAN_POINT ( 'NONE',  ( 47.63139720814400846, -27.50000000000022737, 5.000000000000000888 ) ) ;
#33838=ORIENTED_EDGE ( 'NONE', *, *, #4077, .F. ) ;
#33875=EDGE_CURVE ( 'NONE', #12924, #22186, #16682, .T. ) ;
#34050=ORIENTED_EDGE ( 'NONE', *, *, #13268, .T. ) ;
#34060=ORIENTED_EDGE ( 'NONE', *, *, #20287, .F. ) ;
#34072=CARTESIAN_POINT ( 'NONE',  ( 3.500000000000000888, 55.00000000000000000, -15.00000000000000000 ) ) ;
#34153=ORIENTED_EDGE ( 'NONE', *, *, #3172, .F. ) ;
#34187=ADVANCED_FACE ( 'NONE', ( #24484 ), #33275, .F. ) ;
#34224=ORIENTED_EDGE ( 'NONE', *, *, #16828, .F. ) ;
#34233=DIRECTION ( 'NONE',  ( 0.000000000000000000, 0.000000000000000000, 1.000000000000000000 ) ) ;
#34270=ORIENTED_EDGE ( 'NONE', *, *, #170, .T. ) ;
#34378=VECTOR ( 'NONE', #35092, 1000.000000000000000 ) ;
#34419=CIRCLE ( 'NONE', #3948, 25.00000000000000000 ) ;
#34486=ORIENTED_EDGE ( 'NONE', *, *, #30500, .F. ) ;
#34520=EDGE_CURVE ( 'NONE', #36052, #20938, #22303, .T. ) ;
#34524=FACE_BOUND ( 'NONE', #16363, .T. ) ;
#34591=DIRECTION ( 'NONE',  ( 0.000000000000000000, 0.000000000000000000, 1.000000000000000000 ) ) ;
#34595=CIRCLE ( 'NONE', #20816, 3.500000000000003109 ) ;
#34684=EDGE_LOOP ( 'NONE', ( #1283, #8762, #32878, #421 ) ) ;
#34771=CARTESIAN_POINT ( 'NONE',  ( -45.00000000000000000, 0.000000000000000000, 15.00000000000000000 ) ) ;
#34836=FACE_OUTER_BOUND ( 'NONE', #14583, .T. ) ;
#34869=EDGE_LOOP ( 'NONE', ( #31916, #11442, #34949, #15545, #30965, #11752 ) ) ;
#34882=AXIS2_PLACEMENT_3D ( 'NONE', #17469, #32449, #28885 ) ;
#34943=ORIENTED_EDGE ( 'NONE', *, *, #6873, .T. ) ;
#34949=ORIENTED_EDGE ( 'NONE', *, *, #170, .F. ) ;
#34967=DIRECTION ( 'NONE',  ( 1.000000000000000000, 0.000000000000000000, 0.000000000000000000 ) ) ;
#35092=DIRECTION ( 'NONE',  ( -0.000000000000000000, -0.000000000000000000, 1.000000000000000000 ) ) ;
#35168=CARTESIAN_POINT ( 'NONE',  ( 0.000000000000000000, -55.00000000000000000, -15.00000000000000000 ) ) ;
#35183=EDGE_CURVE ( 'NONE', #14697, #18023, #31281, .T. ) ;
#35196=DIRECTION ( 'NONE',  ( 0.000000000000000000, 0.000000000000000000, 1.000000000000000000 ) ) ;
#35235=DIRECTION ( 'NONE',  ( 0.000000000000000000, 0.000000000000000000, 1.000000000000000000 ) ) ;
#35280=VERTEX_POINT ( 'NONE', #3157 ) ;
#35317=CARTESIAN_POINT ( 'NONE',  ( 0.000000000000000000, 0.000000000000000000, 5.000000000000000000 ) ) ;
#35338=AXIS2_PLACEMENT_3D ( 'NONE', #25072, #33505, #10806 ) ;
#35357=FACE_OUTER_BOUND ( 'NONE', #10363, .T. ) ;
#35372=FACE_OUTER_BOUND ( 'NONE', #19372, .T. ) ;
#35429=ORIENTED_EDGE ( 'NONE', *, *, #14933, .T. ) ;
#35511=ORIENTED_EDGE ( 'NONE', *, *, #4185, .F. ) ;
#35514=CARTESIAN_POINT ( 'NONE',  ( 51.13139720814400846, -27.50000000000022737, 5.000000000000000888 ) ) ;
#35522=ADVANCED_FACE ( 'NONE', ( #15332 ), #7647, .T. ) ;
#35577=DIRECTION ( 'NONE',  ( -0.000000000000000000, -0.000000000000000000, 1.000000000000000000 ) ) ;
#35586=DIRECTION ( 'NONE',  ( 1.000000000000000000, 0.000000000000000000, 0.000000000000000000 ) ) ;
#35631=ORIENTED_EDGE ( 'NONE', *, *, #19302, .F. ) ;
#35638=ORIENTED_EDGE ( 'NONE', *, *, #17219, .F. ) ;
#35649=DIRECTION ( 'NONE',  ( -0.000000000000000000, -0.000000000000000000, 1.000000000000000000 ) ) ;
#35724=EDGE_LOOP ( 'NONE', ( #18719, #6012 ) ) ;
#35749=SURFACE_STYLE_FILL_AREA ( #26929 ) ;
#35780=EDGE_CURVE ( 'NONE', #10920, #24629, #17709, .T. ) ;
#35878=CIRCLE ( 'NONE', #13119, 3.500000000000000888 ) ;
#35898=CARTESIAN_POINT ( 'NONE',  ( 0.000000000000000000, 0.000000000000000000, 15.00000000000000000 ) ) ;
#35916=FACE_OUTER_BOUND ( 'NONE', #15147, .T. ) ;
#35924=DIRECTION ( 'NONE',  ( 1.000000000000000000, 0.000000000000000000, 0.000000000000000000 ) ) ;
#35978=CARTESIAN_POINT ( 'NONE',  ( 0.000000000000000000, 0.000000000000000000, 5.000000000000000000 ) ) ;
#36027=EDGE_CURVE ( 'NONE', #23649, #4478, #28490, .T. ) ;
#36052=VERTEX_POINT ( 'NONE', #30474 ) ;
#36072=CARTESIAN_POINT ( 'NONE',  ( 44.13139720814400135, -27.50000000000022737, 5.000000000000000888 ) ) ;
#36119=DIRECTION ( 'NONE',  ( 1.000000000000000000, 0.000000000000000000, 0.000000000000000000 ) ) ;
#36169=ORIENTED_EDGE ( 'NONE', *, *, #36604, .T. ) ;
#36184=ORIENTED_EDGE ( 'NONE', *, *, #7859, .F. ) ;
#36202=VECTOR ( 'NONE', #19135, 1000.000000000000000 ) ;
#36363=AXIS2_PLACEMENT_3D ( 'NONE', #18470, #9264, #34967 ) ;
#36372=CARTESIAN_POINT ( 'NONE',  ( -44.13139720814380240, 27.50000000000055422, -15.00000000000000000 ) ) ;
#36377=EDGE_LOOP ( 'NONE', ( #20633, #2103 ) ) ;
#36382=DIRECTION ( 'NONE',  ( -0.000000000000000000, -0.000000000000000000, -1.000000000000000000 ) ) ;
#36396=DIRECTION ( 'NONE',  ( 1.000000000000000000, 0.000000000000000000, 0.000000000000000000 ) ) ;
#36430=DIRECTION ( 'NONE',  ( 0.000000000000000000, -0.000000000000000000, 1.000000000000000000 ) ) ;
#36506=ORIENTED_EDGE ( 'NONE', *, *, #36604, .F. ) ;
#36535=AXIS2_PLACEMENT_3D ( 'NONE', #13203, #24648, #15647 ) ;
#36604=EDGE_CURVE ( 'NONE', #24335, #13777, #37062, .T. ) ;
#36689=CARTESIAN_POINT ( 'NONE',  ( 0.000000000000000000, 0.000000000000000000, -15.00000000000000000 ) ) ;
#36696=DIRECTION ( 'NONE',  ( -1.000000000000000000, 0.000000000000000000, 0.000000000000000000 ) ) ;
#36730=CARTESIAN_POINT ( 'NONE',  ( -3.500000000000000888, -55.00000000000000000, 5.000000000000000888 ) ) ;
#36766=DIRECTION ( 'NONE',  ( -0.000000000000000000, -0.000000000000000000, 1.000000000000000000 ) ) ;
#36772=ORIENTED_EDGE ( 'NONE', *, *, #15397, .F. ) ;
#36780=DIRECTION ( 'NONE',  ( 1.000000000000000000, 0.000000000000000000, 0.000000000000000000 ) ) ;
#36808=CARTESIAN_POINT ( 'NONE',  ( 0.000000000000000000, 0.000000000000000000, 15.00000000000000000 ) ) ;
#36827=CIRCLE ( 'NONE', #29634, 3.500000000000000888 ) ;
#36978=FACE_OUTER_BOUND ( 'NONE', #18600, .T. ) ;
#37029=VERTEX_POINT ( 'NONE', #28386 ) ;
#37062=LINE ( 'NONE', #34072, #23149 ) ;
#37076=CARTESIAN_POINT ( 'NONE',  ( 47.63139720814400846, -27.50000000000022737, 5.000000000000000888 ) ) ;
#37086=VECTOR ( 'NONE', #30251, 1000.000000000000000 ) ;
ENDSEC;
END-ISO-10303-21;
